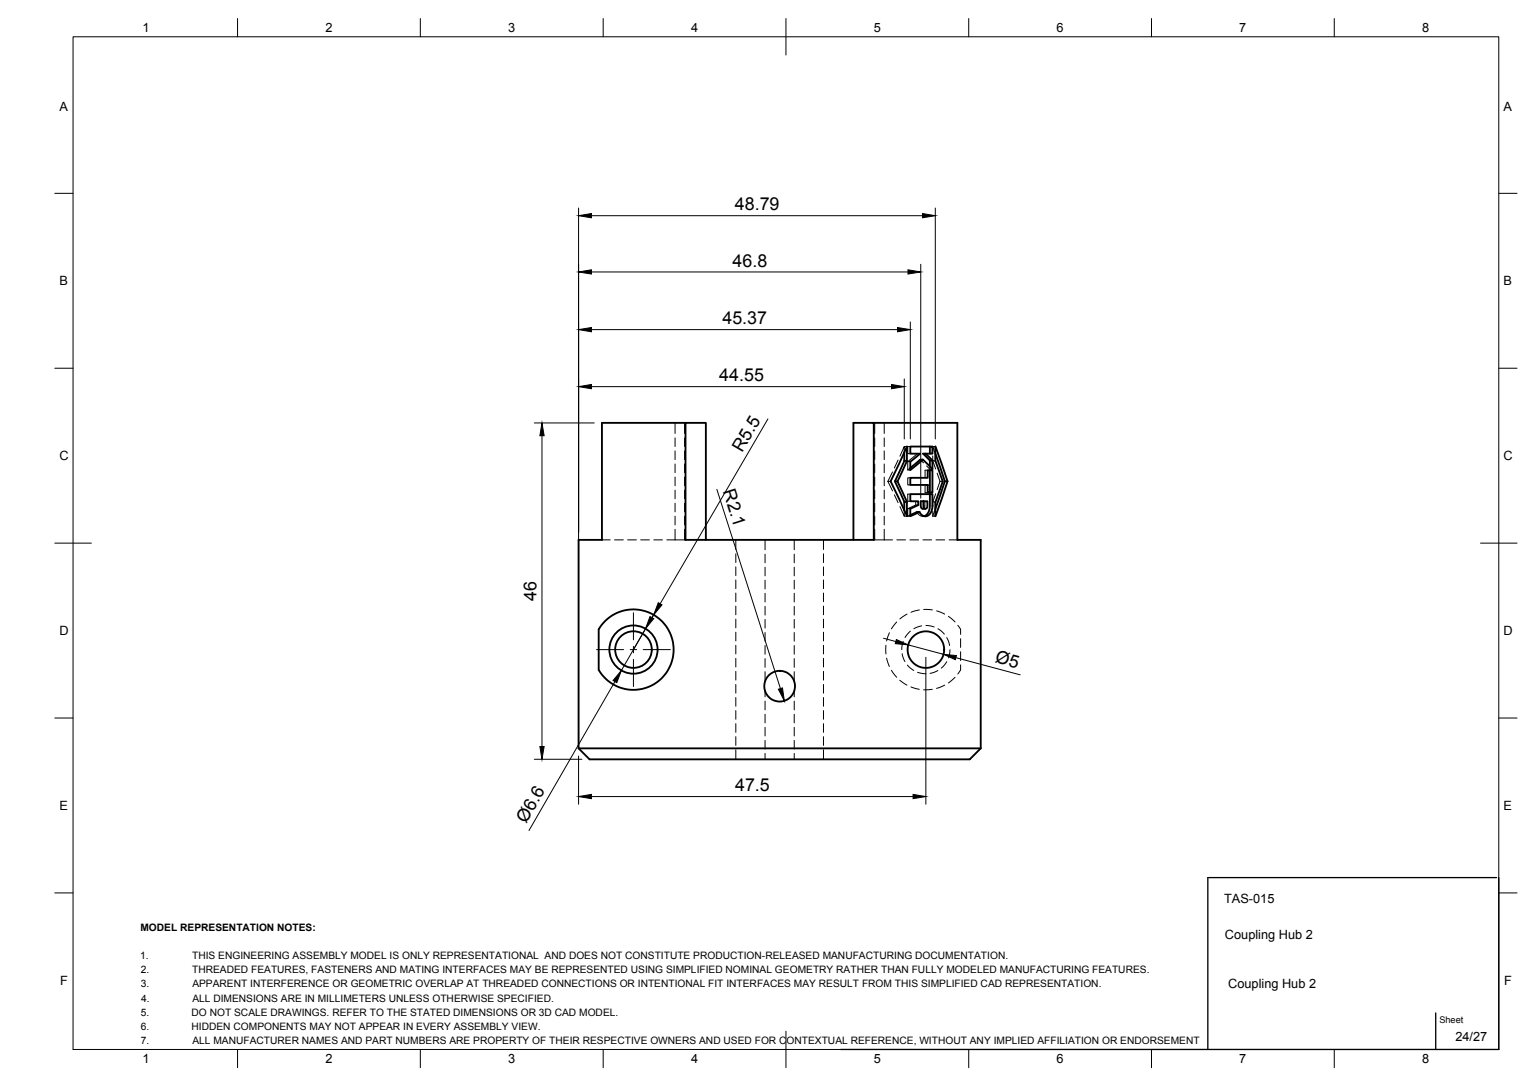
ISO-10303-21;
HEADER;
/* Generated by software containing ST-Developer
 * from STEP Tools, Inc. (www.steptools.com) 
 */

FILE_DESCRIPTION(
/* description */ ('STEP AP214'),
/* implementation_level */ '2;1');

FILE_NAME(
/* name */ 'Coupling Hub 2.step',
/* time_stamp */ '2026-11-15T14:49:54-08:00',
/* author */ (''),
/* organization */ (''),
/* preprocessor_version */ 'ST-DEVELOPER v20.2',
/* originating_system */ 'Autodesk Translation Framework v15.17.0.0',
/* authorisation */ '');

FILE_SCHEMA (('AUTOMOTIVE_DESIGN { 1 0 10303 214 3 1 1 }'));
ENDSEC;

DATA;
#10=MECHANICAL_DESIGN_GEOMETRIC_PRESENTATION_REPRESENTATION('',(#1119,#1120),#66721);
#374=B_SPLINE_CURVE_WITH_KNOTS('',3,(#64255,#64256,#64257,#64258,#64259,
#64260,#64261,#64262,#64263,#64264,#64265,#64266,#64267,#64268,#64269,#64270,
#64271,#64272),.UNSPECIFIED.,.F.,.F.,(4,2,2,2,2,2,2,2,4),(0.567634871268155,
0.624046753014798,0.75751040349095,0.849653931021769,0.941797458552588,
1.03394098608341,1.12608451361423,1.25954816409038,1.39301181456653),
 .UNSPECIFIED.);
#375=B_SPLINE_CURVE_WITH_KNOTS('',3,(#64273,#64274,#64275,#64276,#64277,
#64278,#64279,#64280,#64281,#64282,#64283,#64284,#64285,#64286,#64287,#64288,
#64289,#64290,#64291,#64292,#64293,#64294,#64295,#64296,#64297),
 .UNSPECIFIED.,.F.,.F.,(4,2,2,2,2,3,2,2,2,2,2,4),(1.39301181456653,1.54288207354412,
1.6927523325217,1.78817362481344,1.83588427095931,1.88359491710518,1.93130556325105,
1.97901620939691,2.07443750168865,2.22430776066624,2.37417801964382,2.45122978837333),
 .UNSPECIFIED.);
#376=B_SPLINE_CURVE_WITH_KNOTS('',3,(#64301,#64302,#64303,#64304,#64305,
#64306,#64307,#64308,#64309,#64310,#64311,#64312,#64313,#64314,#64315,#64316,
#64317,#64318,#64319,#64320,#64321,#64322,#64323,#64324,#64325,#64326,#64327,
#64328,#64329,#64330),.UNSPECIFIED.,.F.,.F.,(4,2,2,2,2,2,2,2,2,2,2,2,2,
2,4),(-3.98325608634761,-3.86919217467992,-3.49972652065679,-3.13026086663367,
-2.85088285941717,-2.57150485220067,-2.36940240571059,-2.16729995922052,
-1.96519751273044,-1.76309506624036,-1.48371705902386,-1.20433905180736,
-0.83487339778424,-0.465407743761119,-0.35134383209342),.UNSPECIFIED.);
#377=B_SPLINE_CURVE_WITH_KNOTS('',3,(#64366,#64367,#64368,#64369,#64370,
#64371,#64372,#64373,#64374,#64375,#64376,#64377,#64378,#64379,#64380,#64381,
#64382,#64383,#64384,#64385,#64386,#64387,#64388,#64389,#64390,#64391,#64392,
#64393,#64394,#64395),.UNSPECIFIED.,.F.,.F.,(4,2,2,2,2,2,2,2,2,2,2,2,2,
2,4),(-3.98325608634761,-3.86919217467992,-3.49972652065679,-3.13026086663367,
-2.85088285941717,-2.57150485220067,-2.36940240571059,-2.16729995922052,
-1.96519751273044,-1.76309506624036,-1.48371705902386,-1.20433905180736,
-0.83487339778424,-0.465407743761118,-0.35134383209342),.UNSPECIFIED.);
#378=B_SPLINE_CURVE_WITH_KNOTS('',3,(#64412,#64413,#64414,#64415,#64416,
#64417,#64418,#64419,#64420,#64421,#64422,#64423,#64424,#64425,#64426,#64427,
#64428,#64429,#64430,#64431,#64432,#64433,#64434,#64435,#64436,#64437,#64438,
#64439),.UNSPECIFIED.,.F.,.F.,(4,2,2,2,2,2,2,2,2,2,2,2,2,4),(0.490583102538645,
0.624046753014798,0.75751040349095,0.849653931021769,0.941797458552588,
1.03394098608341,1.12608451361423,1.25954816409038,1.39301181456653,1.54288207354412,
1.6927523325217,1.78817362481344,1.83588427095931,1.88359491710518),
 .UNSPECIFIED.);
#379=B_SPLINE_CURVE_WITH_KNOTS('',3,(#64440,#64441,#64442,#64443,#64444,
#64445,#64446,#64447,#64448,#64449,#64450,#64451),.UNSPECIFIED.,.F.,.F.,
(4,2,2,2,2,4),(0.,0.0477106461458692,0.0954212922917384,0.190842584583477,
0.340712843561061,0.490583102538645),.UNSPECIFIED.);
#380=B_SPLINE_CURVE_WITH_KNOTS('',3,(#64523,#64524,#64525,#64526,#64527,
#64528),.UNSPECIFIED.,.F.,.F.,(4,2,4),(0.575736753726219,0.638728583590876,
0.701720413455533),.UNSPECIFIED.);
#381=B_SPLINE_CURVE_WITH_KNOTS('',3,(#64534,#64535,#64536,#64537,#64538,
#64539,#64540),.UNSPECIFIED.,.F.,.F.,(4,3,4),(-0.0629918298646558,0.,0.0629918298646566),
 .UNSPECIFIED.);
#382=B_SPLINE_CURVE_WITH_KNOTS('',3,(#64547,#64548,#64549,#64550,#64551,
#64552,#64553,#64554,#64555,#64556,#64557,#64558,#64559,#64560,#64561,#64562,
#64563,#64564),.UNSPECIFIED.,.F.,.F.,(4,2,2,2,2,2,2,2,4),(0.,0.0151927838523538,
0.0303855677047076,0.0455818431537581,0.0607781186028086,0.0759788205112384,
0.0911795224196683,0.106372746681134,0.1215659709426),.UNSPECIFIED.);
#383=B_SPLINE_CURVE_WITH_KNOTS('',3,(#64575,#64576,#64577,#64578,#64579,
#64580,#64581,#64582,#64583,#64584,#64585,#64586,#64587,#64588,#64589,#64590,
#64591,#64592),.UNSPECIFIED.,.F.,.F.,(4,2,2,2,2,2,2,2,4),(0.316549052084077,
0.395686269484847,0.474823486885617,0.553960795526886,0.633098104168155,
0.712235412809424,0.791372721450692,0.870509938851462,0.949647156252232),
 .UNSPECIFIED.);
#384=B_SPLINE_CURVE_WITH_KNOTS('',3,(#64594,#64595,#64596,#64597,#64598,
#64599,#64600,#64601,#64602,#64603,#64604,#64605,#64606,#64607,#64608,#64609,
#64610,#64611,#64612,#64613,#64614,#64615,#64616,#64617,#64618,#64619,#64620,
#64621,#64622,#64623,#64624,#64625,#64626,#64627,#64628,#64629,#64630,#64631,
#64632,#64633,#64634,#64635,#64636,#64637,#64638,#64639,#64640,#64641,#64642,
#64643,#64644,#64645,#64646,#64647,#64648,#64649,#64650,#64651,#64652,#64653,
#64654),.UNSPECIFIED.,.F.,.F.,(4,3,3,3,3,3,3,3,3,3,3,3,3,3,3,3,3,3,3,3,
4),(0.,0.0530381009639862,0.106881832368641,0.160741065532074,0.214029097090197,
0.25,0.302729149752815,0.356241665072322,0.409762788184605,0.462708186762728,
0.5,0.552255845605983,0.60528221172878,0.6583187251977,0.710788396881531,
0.75,0.802421738286104,0.855626872469095,0.908846463732818,0.961502691977757,
1.),.UNSPECIFIED.);
#385=B_SPLINE_CURVE_WITH_KNOTS('',3,(#64655,#64656,#64657,#64658,#64659,
#64660,#64661,#64662,#64663,#64664),.UNSPECIFIED.,.F.,.F.,(4,2,2,2,4),(0.949647156252232,
1.028784373653,1.10792159105377,1.18705889969504,1.26619620833631),
 .UNSPECIFIED.);
#386=B_SPLINE_CURVE_WITH_KNOTS('',3,(#64719,#64720,#64721,#64722,#64723,
#64724,#64725,#64726,#64727,#64728,#64729,#64730,#64731,#64732,#64733,#64734),
 .UNSPECIFIED.,.F.,.F.,(4,2,2,2,2,2,2,4),(-0.779703847201594,-0.757646703299412,
-0.7035492015768,-0.649451699854188,-0.595298023055894,-0.5411443462576,
-0.487035463795603,-0.432926581333605),.UNSPECIFIED.);
#387=B_SPLINE_CURVE_WITH_KNOTS('',3,(#64957,#64958,#64959,#64960,#64961,
#64962,#64963,#64964,#64965,#64966,#64967,#64968,#64969,#64970,#64971,#64972),
 .UNSPECIFIED.,.F.,.F.,(4,2,2,2,2,2,2,4),(0.432932407296797,0.487041759940904,
0.541151112585012,0.595306935250484,0.649462757915956,0.703560301016107,
0.757657844116259,0.779715370662846),.UNSPECIFIED.);
#388=B_SPLINE_CURVE_WITH_KNOTS('',3,(#65004,#65005,#65006,#65007,#65008,
#65009,#65010,#65011,#65012,#65013,#65014,#65015,#65016,#65017,#65018,#65019,
#65020,#65021),.UNSPECIFIED.,.F.,.F.,(4,2,2,2,2,2,2,2,4),(0.121566783856533,
0.136760015420318,0.151953246984103,0.167154235901664,0.182355224819225,
0.19755162162294,0.212748018426654,0.22794079306986,0.243133567713066),
 .UNSPECIFIED.);
#553=CONICAL_SURFACE('',#28005,26.75,0.785398163397448);
#554=CONICAL_SURFACE('',#28068,26.75,0.785398163397448);
#658=ELLIPSE('',#28121,54.9999999419771,27.4999999445285);
#659=ELLIPSE('',#28122,55.000000033545,27.5000000336033);
#660=ELLIPSE('',#28123,54.9999999899496,27.4999999902495);
#661=ELLIPSE('',#28124,55.0000000182334,27.5000000177256);
#662=ELLIPSE('',#28125,32.156845610475,27.5);
#663=ELLIPSE('',#28131,33.1709935839343,27.5);
#664=ELLIPSE('',#28132,55.0000000634487,27.5000000626689);
#665=ELLIPSE('',#28133,54.9999999927228,27.4999999930211);
#666=ELLIPSE('',#28134,54.9999999529142,27.4999999544911);
#667=ELLIPSE('',#28135,54.999999883306,27.4999998869508);
#668=ELLIPSE('',#28150,31.5721756903194,27.);
#669=ELLIPSE('',#28153,31.5721756902846,27.);
#670=ELLIPSE('',#28166,32.567884609681,27.);
#671=ELLIPSE('',#28169,54.0000000152791,27.00000001486);
#672=ELLIPSE('',#28170,53.9999998552686,26.9999998599516);
#673=ELLIPSE('',#28171,53.9999996954935,26.9999997042733);
#674=ELLIPSE('',#28172,54.0000000102257,27.0000000099676);
#675=ELLIPSE('',#28181,54.0000000020546,27.0000000020822);
#676=ELLIPSE('',#28183,53.9999999941722,26.9999999944392);
#677=ELLIPSE('',#28186,54.0000000784931,27.0000000775048);
#678=ELLIPSE('',#28188,54.0000000505798,27.0000000505259);
#1057=SHAPE_REPRESENTATION_RELATIONSHIP('SRR','None',#66920,#1088);
#1088=ADVANCED_BREP_SHAPE_REPRESENTATION('',(#1154,#1155),#66711);
#1119=STYLED_ITEM('',(#67095),#1154);
#1120=STYLED_ITEM('',(#67095),#1155);
#1154=MANIFOLD_SOLID_BREP('Body1',#25685);
#1155=MANIFOLD_SOLID_BREP('Body2',#25686);
#1408=FACE_BOUND('',#5046,.T.);
#1409=FACE_BOUND('',#5047,.T.);
#1410=FACE_BOUND('',#5052,.T.);
#1411=FACE_BOUND('',#5055,.T.);
#1412=FACE_BOUND('',#5058,.T.);
#1413=FACE_BOUND('',#5060,.T.);
#1414=FACE_BOUND('',#5064,.T.);
#1415=FACE_BOUND('',#5068,.T.);
#1416=FACE_BOUND('',#5071,.T.);
#1417=FACE_BOUND('',#5073,.T.);
#1418=FACE_BOUND('',#5096,.T.);
#1419=FACE_BOUND('',#5097,.T.);
#1420=FACE_BOUND('',#5098,.T.);
#1421=FACE_BOUND('',#5099,.T.);
#1422=FACE_BOUND('',#5100,.T.);
#1423=FACE_BOUND('',#5101,.T.);
#1424=FACE_BOUND('',#5102,.T.);
#1425=FACE_BOUND('',#5103,.T.);
#1426=FACE_BOUND('',#5153,.T.);
#2055=PLANE('',#28002);
#2056=PLANE('',#28007);
#2057=PLANE('',#28012);
#2058=PLANE('',#28035);
#2059=PLANE('',#28038);
#2060=PLANE('',#28043);
#2061=PLANE('',#28047);
#2062=PLANE('',#28048);
#2063=PLANE('',#28052);
#2064=PLANE('',#28058);
#2065=PLANE('',#28062);
#2066=PLANE('',#28063);
#2067=PLANE('',#28064);
#2068=PLANE('',#28070);
#2069=PLANE('',#28090);
#2070=PLANE('',#28091);
#2071=PLANE('',#28092);
#2072=PLANE('',#28093);
#2073=PLANE('',#28094);
#2074=PLANE('',#28095);
#2075=PLANE('',#28108);
#2076=PLANE('',#28110);
#2077=PLANE('',#28141);
#2078=PLANE('',#28142);
#2079=PLANE('',#28143);
#2080=PLANE('',#28144);
#2081=PLANE('',#28145);
#2082=PLANE('',#28146);
#2083=PLANE('',#28147);
#2084=PLANE('',#28148);
#2085=PLANE('',#28149);
#2086=PLANE('',#28151);
#2087=PLANE('',#28152);
#2088=PLANE('',#28154);
#2089=PLANE('',#28155);
#2090=PLANE('',#28157);
#2091=PLANE('',#28159);
#2092=PLANE('',#28160);
#2093=PLANE('',#28162);
#2094=PLANE('',#28163);
#2095=PLANE('',#28165);
#2096=PLANE('',#28173);
#2097=PLANE('',#28174);
#2098=PLANE('',#28175);
#2099=PLANE('',#28176);
#2100=PLANE('',#28177);
#2101=PLANE('',#28178);
#2102=PLANE('',#28179);
#2103=PLANE('',#28180);
#2104=PLANE('',#28182);
#2105=PLANE('',#28184);
#2106=PLANE('',#28185);
#2107=PLANE('',#28187);
#2108=PLANE('',#28190);
#2109=PLANE('',#28192);
#2110=PLANE('',#28193);
#2111=PLANE('',#28196);
#2112=PLANE('',#28197);
#2113=PLANE('',#28199);
#2114=PLANE('',#28200);
#2115=PLANE('',#28202);
#2116=PLANE('',#28203);
#2117=PLANE('',#28205);
#2118=PLANE('',#28207);
#3353=FACE_OUTER_BOUND('',#5035,.T.);
#3354=FACE_OUTER_BOUND('',#5036,.T.);
#3355=FACE_OUTER_BOUND('',#5037,.T.);
#3356=FACE_OUTER_BOUND('',#5038,.T.);
#3357=FACE_OUTER_BOUND('',#5039,.T.);
#3358=FACE_OUTER_BOUND('',#5040,.T.);
#3359=FACE_OUTER_BOUND('',#5041,.T.);
#3360=FACE_OUTER_BOUND('',#5042,.T.);
#3361=FACE_OUTER_BOUND('',#5043,.T.);
#3362=FACE_OUTER_BOUND('',#5044,.T.);
#3363=FACE_OUTER_BOUND('',#5045,.T.);
#3364=FACE_OUTER_BOUND('',#5048,.T.);
#3365=FACE_OUTER_BOUND('',#5049,.T.);
#3366=FACE_OUTER_BOUND('',#5050,.T.);
#3367=FACE_OUTER_BOUND('',#5051,.T.);
#3368=FACE_OUTER_BOUND('',#5053,.T.);
#3369=FACE_OUTER_BOUND('',#5054,.T.);
#3370=FACE_OUTER_BOUND('',#5056,.T.);
#3371=FACE_OUTER_BOUND('',#5057,.T.);
#3372=FACE_OUTER_BOUND('',#5059,.T.);
#3373=FACE_OUTER_BOUND('',#5061,.T.);
#3374=FACE_OUTER_BOUND('',#5062,.T.);
#3375=FACE_OUTER_BOUND('',#5063,.T.);
#3376=FACE_OUTER_BOUND('',#5065,.T.);
#3377=FACE_OUTER_BOUND('',#5066,.T.);
#3378=FACE_OUTER_BOUND('',#5067,.T.);
#3379=FACE_OUTER_BOUND('',#5069,.T.);
#3380=FACE_OUTER_BOUND('',#5070,.T.);
#3381=FACE_OUTER_BOUND('',#5072,.T.);
#3382=FACE_OUTER_BOUND('',#5074,.T.);
#3383=FACE_OUTER_BOUND('',#5075,.T.);
#3384=FACE_OUTER_BOUND('',#5076,.T.);
#3385=FACE_OUTER_BOUND('',#5077,.T.);
#3386=FACE_OUTER_BOUND('',#5078,.T.);
#3387=FACE_OUTER_BOUND('',#5079,.T.);
#3388=FACE_OUTER_BOUND('',#5080,.T.);
#3389=FACE_OUTER_BOUND('',#5081,.T.);
#3390=FACE_OUTER_BOUND('',#5082,.T.);
#3391=FACE_OUTER_BOUND('',#5083,.T.);
#3392=FACE_OUTER_BOUND('',#5084,.T.);
#3393=FACE_OUTER_BOUND('',#5085,.T.);
#3394=FACE_OUTER_BOUND('',#5086,.T.);
#3395=FACE_OUTER_BOUND('',#5087,.T.);
#3396=FACE_OUTER_BOUND('',#5088,.T.);
#3397=FACE_OUTER_BOUND('',#5089,.T.);
#3398=FACE_OUTER_BOUND('',#5090,.T.);
#3399=FACE_OUTER_BOUND('',#5091,.T.);
#3400=FACE_OUTER_BOUND('',#5092,.T.);
#3401=FACE_OUTER_BOUND('',#5093,.T.);
#3402=FACE_OUTER_BOUND('',#5094,.T.);
#3403=FACE_OUTER_BOUND('',#5095,.T.);
#3404=FACE_OUTER_BOUND('',#5104,.T.);
#3405=FACE_OUTER_BOUND('',#5105,.T.);
#3406=FACE_OUTER_BOUND('',#5106,.T.);
#3407=FACE_OUTER_BOUND('',#5107,.T.);
#3408=FACE_OUTER_BOUND('',#5108,.T.);
#3409=FACE_OUTER_BOUND('',#5109,.T.);
#3410=FACE_OUTER_BOUND('',#5110,.T.);
#3411=FACE_OUTER_BOUND('',#5111,.T.);
#3412=FACE_OUTER_BOUND('',#5112,.T.);
#3413=FACE_OUTER_BOUND('',#5113,.T.);
#3414=FACE_OUTER_BOUND('',#5114,.T.);
#3415=FACE_OUTER_BOUND('',#5115,.T.);
#3416=FACE_OUTER_BOUND('',#5116,.T.);
#3417=FACE_OUTER_BOUND('',#5117,.T.);
#3418=FACE_OUTER_BOUND('',#5118,.T.);
#3419=FACE_OUTER_BOUND('',#5119,.T.);
#3420=FACE_OUTER_BOUND('',#5120,.T.);
#3421=FACE_OUTER_BOUND('',#5121,.T.);
#3422=FACE_OUTER_BOUND('',#5122,.T.);
#3423=FACE_OUTER_BOUND('',#5123,.T.);
#3424=FACE_OUTER_BOUND('',#5124,.T.);
#3425=FACE_OUTER_BOUND('',#5125,.T.);
#3426=FACE_OUTER_BOUND('',#5126,.T.);
#3427=FACE_OUTER_BOUND('',#5127,.T.);
#3428=FACE_OUTER_BOUND('',#5128,.T.);
#3429=FACE_OUTER_BOUND('',#5129,.T.);
#3430=FACE_OUTER_BOUND('',#5130,.T.);
#3431=FACE_OUTER_BOUND('',#5131,.T.);
#3432=FACE_OUTER_BOUND('',#5132,.T.);
#3433=FACE_OUTER_BOUND('',#5133,.T.);
#3434=FACE_OUTER_BOUND('',#5134,.T.);
#3435=FACE_OUTER_BOUND('',#5135,.T.);
#3436=FACE_OUTER_BOUND('',#5136,.T.);
#3437=FACE_OUTER_BOUND('',#5137,.T.);
#3438=FACE_OUTER_BOUND('',#5138,.T.);
#3439=FACE_OUTER_BOUND('',#5139,.T.);
#3440=FACE_OUTER_BOUND('',#5140,.T.);
#3441=FACE_OUTER_BOUND('',#5141,.T.);
#3442=FACE_OUTER_BOUND('',#5142,.T.);
#3443=FACE_OUTER_BOUND('',#5143,.T.);
#3444=FACE_OUTER_BOUND('',#5144,.T.);
#3445=FACE_OUTER_BOUND('',#5145,.T.);
#3446=FACE_OUTER_BOUND('',#5146,.T.);
#3447=FACE_OUTER_BOUND('',#5147,.T.);
#3448=FACE_OUTER_BOUND('',#5148,.T.);
#3449=FACE_OUTER_BOUND('',#5149,.T.);
#3450=FACE_OUTER_BOUND('',#5150,.T.);
#3451=FACE_OUTER_BOUND('',#5151,.T.);
#3452=FACE_OUTER_BOUND('',#5152,.T.);
#5035=EDGE_LOOP('',(#22080,#22081,#22082,#22083));
#5036=EDGE_LOOP('',(#22084,#22085,#22086,#22087));
#5037=EDGE_LOOP('',(#22088,#22089,#22090,#22091));
#5038=EDGE_LOOP('',(#22092,#22093,#22094,#22095));
#5039=EDGE_LOOP('',(#22096,#22097,#22098,#22099));
#5040=EDGE_LOOP('',(#22100,#22101,#22102,#22103));
#5041=EDGE_LOOP('',(#22104,#22105,#22106,#22107));
#5042=EDGE_LOOP('',(#22108,#22109,#22110,#22111));
#5043=EDGE_LOOP('',(#22112,#22113,#22114,#22115));
#5044=EDGE_LOOP('',(#22116,#22117,#22118,#22119));
#5045=EDGE_LOOP('',(#22120,#22121,#22122,#22123,#22124,#22125,#22126,#22127,
#22128,#22129,#22130,#22131));
#5046=EDGE_LOOP('',(#22132,#22133));
#5047=EDGE_LOOP('',(#22134,#22135));
#5048=EDGE_LOOP('',(#22136,#22137,#22138,#22139));
#5049=EDGE_LOOP('',(#22140,#22141,#22142,#22143,#22144,#22145,#22146,#22147,
#22148,#22149,#22150,#22151));
#5050=EDGE_LOOP('',(#22152,#22153,#22154,#22155,#22156));
#5051=EDGE_LOOP('',(#22157,#22158));
#5052=EDGE_LOOP('',(#22159));
#5053=EDGE_LOOP('',(#22160,#22161,#22162,#22163));
#5054=EDGE_LOOP('',(#22164));
#5055=EDGE_LOOP('',(#22165));
#5056=EDGE_LOOP('',(#22166,#22167,#22168,#22169));
#5057=EDGE_LOOP('',(#22170,#22171,#22172,#22173,#22174));
#5058=EDGE_LOOP('',(#22175));
#5059=EDGE_LOOP('',(#22176,#22177,#22178,#22179,#22180));
#5060=EDGE_LOOP('',(#22181));
#5061=EDGE_LOOP('',(#22182,#22183));
#5062=EDGE_LOOP('',(#22184,#22185));
#5063=EDGE_LOOP('',(#22186,#22187,#22188,#22189,#22190));
#5064=EDGE_LOOP('',(#22191));
#5065=EDGE_LOOP('',(#22192,#22193,#22194,#22195,#22196));
#5066=EDGE_LOOP('',(#22197,#22198,#22199,#22200));
#5067=EDGE_LOOP('',(#22201));
#5068=EDGE_LOOP('',(#22202));
#5069=EDGE_LOOP('',(#22203,#22204,#22205,#22206));
#5070=EDGE_LOOP('',(#22207,#22208));
#5071=EDGE_LOOP('',(#22209));
#5072=EDGE_LOOP('',(#22210,#22211,#22212,#22213,#22214));
#5073=EDGE_LOOP('',(#22215));
#5074=EDGE_LOOP('',(#22216,#22217,#22218,#22219,#22220,#22221,#22222,#22223));
#5075=EDGE_LOOP('',(#22224,#22225,#22226,#22227));
#5076=EDGE_LOOP('',(#22228,#22229,#22230,#22231,#22232,#22233,#22234,#22235,
#22236,#22237,#22238,#22239,#22240,#22241,#22242,#22243));
#5077=EDGE_LOOP('',(#22244,#22245,#22246,#22247,#22248,#22249));
#5078=EDGE_LOOP('',(#22250,#22251,#22252,#22253,#22254,#22255));
#5079=EDGE_LOOP('',(#22256,#22257,#22258,#22259));
#5080=EDGE_LOOP('',(#22260,#22261,#22262,#22263,#22264,#22265,#22266,#22267,
#22268,#22269,#22270,#22271,#22272,#22273));
#5081=EDGE_LOOP('',(#22274,#22275,#22276,#22277));
#5082=EDGE_LOOP('',(#22278,#22279,#22280,#22281));
#5083=EDGE_LOOP('',(#22282,#22283,#22284,#22285,#22286));
#5084=EDGE_LOOP('',(#22287,#22288,#22289,#22290));
#5085=EDGE_LOOP('',(#22291,#22292,#22293,#22294));
#5086=EDGE_LOOP('',(#22295,#22296,#22297,#22298));
#5087=EDGE_LOOP('',(#22299,#22300,#22301,#22302));
#5088=EDGE_LOOP('',(#22303,#22304,#22305,#22306));
#5089=EDGE_LOOP('',(#22307,#22308,#22309,#22310));
#5090=EDGE_LOOP('',(#22311,#22312,#22313,#22314));
#5091=EDGE_LOOP('',(#22315,#22316,#22317,#22318));
#5092=EDGE_LOOP('',(#22319,#22320,#22321,#22322));
#5093=EDGE_LOOP('',(#22323,#22324,#22325,#22326));
#5094=EDGE_LOOP('',(#22327,#22328,#22329,#22330));
#5095=EDGE_LOOP('',(#22331,#22332,#22333,#22334,#22335,#22336,#22337,#22338,
#22339,#22340,#22341,#22342));
#5096=EDGE_LOOP('',(#22343,#22344));
#5097=EDGE_LOOP('',(#22345,#22346,#22347,#22348,#22349,#22350,#22351,#22352,
#22353));
#5098=EDGE_LOOP('',(#22354,#22355,#22356,#22357,#22358,#22359,#22360,#22361));
#5099=EDGE_LOOP('',(#22362,#22363,#22364));
#5100=EDGE_LOOP('',(#22365,#22366));
#5101=EDGE_LOOP('',(#22367,#22368,#22369,#22370,#22371,#22372));
#5102=EDGE_LOOP('',(#22373,#22374,#22375,#22376,#22377,#22378,#22379,#22380,
#22381,#22382,#22383));
#5103=EDGE_LOOP('',(#22384,#22385,#22386,#22387,#22388,#22389));
#5104=EDGE_LOOP('',(#22390,#22391,#22392,#22393,#22394,#22395,#22396,#22397));
#5105=EDGE_LOOP('',(#22398,#22399,#22400,#22401));
#5106=EDGE_LOOP('',(#22402,#22403,#22404,#22405));
#5107=EDGE_LOOP('',(#22406,#22407,#22408,#22409));
#5108=EDGE_LOOP('',(#22410,#22411,#22412,#22413));
#5109=EDGE_LOOP('',(#22414,#22415,#22416,#22417));
#5110=EDGE_LOOP('',(#22418,#22419,#22420,#22421));
#5111=EDGE_LOOP('',(#22422,#22423,#22424,#22425));
#5112=EDGE_LOOP('',(#22426,#22427,#22428,#22429));
#5113=EDGE_LOOP('',(#22430,#22431,#22432,#22433));
#5114=EDGE_LOOP('',(#22434,#22435,#22436,#22437));
#5115=EDGE_LOOP('',(#22438,#22439,#22440,#22441));
#5116=EDGE_LOOP('',(#22442,#22443,#22444,#22445));
#5117=EDGE_LOOP('',(#22446,#22447,#22448,#22449));
#5118=EDGE_LOOP('',(#22450,#22451,#22452,#22453));
#5119=EDGE_LOOP('',(#22454,#22455,#22456,#22457));
#5120=EDGE_LOOP('',(#22458,#22459,#22460,#22461));
#5121=EDGE_LOOP('',(#22462,#22463,#22464,#22465));
#5122=EDGE_LOOP('',(#22466,#22467,#22468,#22469));
#5123=EDGE_LOOP('',(#22470,#22471,#22472,#22473));
#5124=EDGE_LOOP('',(#22474,#22475,#22476,#22477,#22478,#22479,#22480,#22481,
#22482,#22483,#22484));
#5125=EDGE_LOOP('',(#22485,#22486,#22487,#22488,#22489,#22490));
#5126=EDGE_LOOP('',(#22491,#22492,#22493,#22494));
#5127=EDGE_LOOP('',(#22495,#22496,#22497,#22498));
#5128=EDGE_LOOP('',(#22499,#22500,#22501,#22502));
#5129=EDGE_LOOP('',(#22503,#22504,#22505,#22506));
#5130=EDGE_LOOP('',(#22507,#22508,#22509,#22510));
#5131=EDGE_LOOP('',(#22511,#22512,#22513,#22514));
#5132=EDGE_LOOP('',(#22515,#22516,#22517,#22518));
#5133=EDGE_LOOP('',(#22519,#22520,#22521,#22522));
#5134=EDGE_LOOP('',(#22523,#22524,#22525,#22526));
#5135=EDGE_LOOP('',(#22527,#22528,#22529,#22530));
#5136=EDGE_LOOP('',(#22531,#22532,#22533,#22534));
#5137=EDGE_LOOP('',(#22535,#22536,#22537,#22538));
#5138=EDGE_LOOP('',(#22539,#22540,#22541,#22542,#22543,#22544));
#5139=EDGE_LOOP('',(#22545,#22546,#22547,#22548));
#5140=EDGE_LOOP('',(#22549,#22550,#22551,#22552));
#5141=EDGE_LOOP('',(#22553,#22554,#22555,#22556));
#5142=EDGE_LOOP('',(#22557,#22558,#22559,#22560));
#5143=EDGE_LOOP('',(#22561,#22562,#22563,#22564));
#5144=EDGE_LOOP('',(#22565,#22566,#22567,#22568));
#5145=EDGE_LOOP('',(#22569,#22570,#22571,#22572));
#5146=EDGE_LOOP('',(#22573,#22574,#22575,#22576));
#5147=EDGE_LOOP('',(#22577,#22578,#22579,#22580));
#5148=EDGE_LOOP('',(#22581,#22582,#22583,#22584));
#5149=EDGE_LOOP('',(#22585,#22586,#22587,#22588));
#5150=EDGE_LOOP('',(#22589,#22590,#22591,#22592));
#5151=EDGE_LOOP('',(#22593,#22594,#22595,#22596));
#5152=EDGE_LOOP('',(#22597,#22598,#22599,#22600,#22601,#22602,#22603,#22604,
#22605));
#5153=EDGE_LOOP('',(#22606,#22607,#22608,#22609));
#6962=LINE('',#64187,#8951);
#6963=LINE('',#64191,#8952);
#6964=LINE('',#64197,#8953);
#6965=LINE('',#64198,#8954);
#6966=LINE('',#64221,#8955);
#6967=LINE('',#64222,#8956);
#6968=LINE('',#64225,#8957);
#6969=LINE('',#64227,#8958);
#6970=LINE('',#64231,#8959);
#6971=LINE('',#64235,#8960);
#6972=LINE('',#64240,#8961);
#6973=LINE('',#64244,#8962);
#6974=LINE('',#64249,#8963);
#6975=LINE('',#64251,#8964);
#6976=LINE('',#64300,#8965);
#6977=LINE('',#64333,#8966);
#6978=LINE('',#64336,#8967);
#6979=LINE('',#64338,#8968);
#6980=LINE('',#64339,#8969);
#6981=LINE('',#64342,#8970);
#6982=LINE('',#64351,#8971);
#6983=LINE('',#64358,#8972);
#6984=LINE('',#64399,#8973);
#6985=LINE('',#64401,#8974);
#6986=LINE('',#64403,#8975);
#6987=LINE('',#64405,#8976);
#6988=LINE('',#64406,#8977);
#6989=LINE('',#64452,#8978);
#6990=LINE('',#64457,#8979);
#6991=LINE('',#64464,#8980);
#6992=LINE('',#64467,#8981);
#6993=LINE('',#64471,#8982);
#6994=LINE('',#64473,#8983);
#6995=LINE('',#64475,#8984);
#6996=LINE('',#64477,#8985);
#6997=LINE('',#64478,#8986);
#6998=LINE('',#64483,#8987);
#6999=LINE('',#64485,#8988);
#7000=LINE('',#64487,#8989);
#7001=LINE('',#64513,#8990);
#7002=LINE('',#64515,#8991);
#7003=LINE('',#64517,#8992);
#7004=LINE('',#64521,#8993);
#7005=LINE('',#64529,#8994);
#7006=LINE('',#64532,#8995);
#7007=LINE('',#64541,#8996);
#7008=LINE('',#64545,#8997);
#7009=LINE('',#64566,#8998);
#7010=LINE('',#64573,#8999);
#7011=LINE('',#64667,#9000);
#7012=LINE('',#64669,#9001);
#7013=LINE('',#64672,#9002);
#7014=LINE('',#64673,#9003);
#7015=LINE('',#64675,#9004);
#7016=LINE('',#64677,#9005);
#7017=LINE('',#64679,#9006);
#7018=LINE('',#64681,#9007);
#7019=LINE('',#64688,#9008);
#7020=LINE('',#64689,#9009);
#7021=LINE('',#64694,#9010);
#7022=LINE('',#64695,#9011);
#7023=LINE('',#64698,#9012);
#7024=LINE('',#64701,#9013);
#7025=LINE('',#64705,#9014);
#7026=LINE('',#64710,#9015);
#7027=LINE('',#64738,#9016);
#7028=LINE('',#64742,#9017);
#7029=LINE('',#64746,#9018);
#7030=LINE('',#64749,#9019);
#7031=LINE('',#64754,#9020);
#7032=LINE('',#64758,#9021);
#7033=LINE('',#64762,#9022);
#7034=LINE('',#64765,#9023);
#7035=LINE('',#64768,#9024);
#7036=LINE('',#64774,#9025);
#7037=LINE('',#64782,#9026);
#7038=LINE('',#64788,#9027);
#7039=LINE('',#64792,#9028);
#7040=LINE('',#64798,#9029);
#7041=LINE('',#64804,#9030);
#7042=LINE('',#64810,#9031);
#7043=LINE('',#64817,#9032);
#7044=LINE('',#64821,#9033);
#7045=LINE('',#64825,#9034);
#7046=LINE('',#64828,#9035);
#7047=LINE('',#64830,#9036);
#7048=LINE('',#64831,#9037);
#7049=LINE('',#64833,#9038);
#7050=LINE('',#64835,#9039);
#7051=LINE('',#64837,#9040);
#7052=LINE('',#64839,#9041);
#7053=LINE('',#64841,#9042);
#7054=LINE('',#64843,#9043);
#7055=LINE('',#64847,#9044);
#7056=LINE('',#64850,#9045);
#7057=LINE('',#64853,#9046);
#7058=LINE('',#64854,#9047);
#7059=LINE('',#64857,#9048);
#7060=LINE('',#64861,#9049);
#7061=LINE('',#64863,#9050);
#7062=LINE('',#64864,#9051);
#7063=LINE('',#64867,#9052);
#7064=LINE('',#64871,#9053);
#7065=LINE('',#64875,#9054);
#7066=LINE('',#64876,#9055);
#7067=LINE('',#64879,#9056);
#7068=LINE('',#64883,#9057);
#7069=LINE('',#64884,#9058);
#7070=LINE('',#64895,#9059);
#7071=LINE('',#64901,#9060);
#7072=LINE('',#64904,#9061);
#7073=LINE('',#64905,#9062);
#7074=LINE('',#64907,#9063);
#7075=LINE('',#64909,#9064);
#7076=LINE('',#64911,#9065);
#7077=LINE('',#64913,#9066);
#7078=LINE('',#64917,#9067);
#7079=LINE('',#64919,#9068);
#7080=LINE('',#64920,#9069);
#7081=LINE('',#64923,#9070);
#7082=LINE('',#64927,#9071);
#7083=LINE('',#64931,#9072);
#7084=LINE('',#64932,#9073);
#7085=LINE('',#64936,#9074);
#7086=LINE('',#64942,#9075);
#7087=LINE('',#64945,#9076);
#7088=LINE('',#64948,#9077);
#7089=LINE('',#64949,#9078);
#7090=LINE('',#64952,#9079);
#7091=LINE('',#64956,#9080);
#7092=LINE('',#64975,#9081);
#7093=LINE('',#64976,#9082);
#7094=LINE('',#64979,#9083);
#7095=LINE('',#64982,#9084);
#7096=LINE('',#64985,#9085);
#7097=LINE('',#64986,#9086);
#7098=LINE('',#64989,#9087);
#7099=LINE('',#64993,#9088);
#7100=LINE('',#64994,#9089);
#7101=LINE('',#64997,#9090);
#7102=LINE('',#65000,#9091);
#7103=LINE('',#65003,#9092);
#7104=LINE('',#65023,#9093);
#8951=VECTOR('',#34159,1000.);
#8952=VECTOR('',#34162,1000.);
#8953=VECTOR('',#34169,1000.);
#8954=VECTOR('',#34170,1000.);
#8955=VECTOR('',#34195,1000.);
#8956=VECTOR('',#34196,1000.);
#8957=VECTOR('',#34199,1000.);
#8958=VECTOR('',#34200,1000.);
#8959=VECTOR('',#34205,1000.);
#8960=VECTOR('',#34210,1000.);
#8961=VECTOR('',#34217,1000.);
#8962=VECTOR('',#34222,1000.);
#8963=VECTOR('',#34229,1000.);
#8964=VECTOR('',#34230,1000.);
#8965=VECTOR('',#34233,1000.);
#8966=VECTOR('',#34236,1000.);
#8967=VECTOR('',#34239,1000.);
#8968=VECTOR('',#34242,1000.);
#8969=VECTOR('',#34243,1000.);
#8970=VECTOR('',#34246,2.5);
#8971=VECTOR('',#34259,3.3);
#8972=VECTOR('',#34268,2.5);
#8973=VECTOR('',#34281,1000.);
#8974=VECTOR('',#34282,1000.);
#8975=VECTOR('',#34283,1000.);
#8976=VECTOR('',#34284,1000.);
#8977=VECTOR('',#34285,1000.);
#8978=VECTOR('',#34290,2.5);
#8979=VECTOR('',#34295,2.5);
#8980=VECTOR('',#34304,3.3);
#8981=VECTOR('',#34309,1000.);
#8982=VECTOR('',#34312,1000.);
#8983=VECTOR('',#34313,1000.);
#8984=VECTOR('',#34314,1000.);
#8985=VECTOR('',#34315,1000.);
#8986=VECTOR('',#34316,1000.);
#8987=VECTOR('',#34321,1000.);
#8988=VECTOR('',#34322,1000.);
#8989=VECTOR('',#34323,1000.);
#8990=VECTOR('',#34354,1000.);
#8991=VECTOR('',#34355,1000.);
#8992=VECTOR('',#34356,1000.);
#8993=VECTOR('',#34361,1000.);
#8994=VECTOR('',#34362,1000.);
#8995=VECTOR('',#34365,1000.);
#8996=VECTOR('',#34366,1000.);
#8997=VECTOR('',#34369,1000.);
#8998=VECTOR('',#34370,1000.);
#8999=VECTOR('',#34377,2.1);
#9000=VECTOR('',#34380,1000.);
#9001=VECTOR('',#34381,1000.);
#9002=VECTOR('',#34384,1000.);
#9003=VECTOR('',#34385,1000.);
#9004=VECTOR('',#34388,1000.);
#9005=VECTOR('',#34391,1000.);
#9006=VECTOR('',#34394,1000.);
#9007=VECTOR('',#34397,1000.);
#9008=VECTOR('',#34406,1000.);
#9009=VECTOR('',#34407,1000.);
#9010=VECTOR('',#34412,1000.);
#9011=VECTOR('',#34413,1000.);
#9012=VECTOR('',#34416,1000.);
#9013=VECTOR('',#34419,1000.);
#9014=VECTOR('',#34424,1000.);
#9015=VECTOR('',#34431,1000.);
#9016=VECTOR('',#34446,1000.);
#9017=VECTOR('',#34449,1000.);
#9018=VECTOR('',#34452,1000.);
#9019=VECTOR('',#34455,1000.);
#9020=VECTOR('',#34458,1000.);
#9021=VECTOR('',#34461,1000.);
#9022=VECTOR('',#34464,1000.);
#9023=VECTOR('',#34467,1000.);
#9024=VECTOR('',#34468,1000.);
#9025=VECTOR('',#34473,1000.);
#9026=VECTOR('',#34480,1000.);
#9027=VECTOR('',#34485,1000.);
#9028=VECTOR('',#34488,1000.);
#9029=VECTOR('',#34493,1000.);
#9030=VECTOR('',#34498,1000.);
#9031=VECTOR('',#34503,1000.);
#9032=VECTOR('',#34510,1000.);
#9033=VECTOR('',#34513,1000.);
#9034=VECTOR('',#34516,1000.);
#9035=VECTOR('',#34519,1000.);
#9036=VECTOR('',#34522,1000.);
#9037=VECTOR('',#34523,1000.);
#9038=VECTOR('',#34526,1000.);
#9039=VECTOR('',#34529,1000.);
#9040=VECTOR('',#34532,1000.);
#9041=VECTOR('',#34535,1000.);
#9042=VECTOR('',#34538,1000.);
#9043=VECTOR('',#34541,1000.);
#9044=VECTOR('',#34546,1000.);
#9045=VECTOR('',#34549,1000.);
#9046=VECTOR('',#34552,1000.);
#9047=VECTOR('',#34553,1000.);
#9048=VECTOR('',#34556,1000.);
#9049=VECTOR('',#34561,1000.);
#9050=VECTOR('',#34562,1000.);
#9051=VECTOR('',#34563,1000.);
#9052=VECTOR('',#34566,1000.);
#9053=VECTOR('',#34571,1000.);
#9054=VECTOR('',#34576,1000.);
#9055=VECTOR('',#34577,1000.);
#9056=VECTOR('',#34580,1000.);
#9057=VECTOR('',#34585,1000.);
#9058=VECTOR('',#34586,1000.);
#9059=VECTOR('',#34601,1000.);
#9060=VECTOR('',#34606,1000.);
#9061=VECTOR('',#34611,1000.);
#9062=VECTOR('',#34612,1000.);
#9063=VECTOR('',#34615,1000.);
#9064=VECTOR('',#34618,1000.);
#9065=VECTOR('',#34621,1000.);
#9066=VECTOR('',#34624,1000.);
#9067=VECTOR('',#34629,1000.);
#9068=VECTOR('',#34630,1000.);
#9069=VECTOR('',#34631,1000.);
#9070=VECTOR('',#34634,1000.);
#9071=VECTOR('',#34639,1000.);
#9072=VECTOR('',#34644,1000.);
#9073=VECTOR('',#34645,1000.);
#9074=VECTOR('',#34650,1000.);
#9075=VECTOR('',#34659,1000.);
#9076=VECTOR('',#34662,1000.);
#9077=VECTOR('',#34665,1000.);
#9078=VECTOR('',#34666,1000.);
#9079=VECTOR('',#34669,1000.);
#9080=VECTOR('',#34674,1000.);
#9081=VECTOR('',#34677,1000.);
#9082=VECTOR('',#34678,1000.);
#9083=VECTOR('',#34681,1000.);
#9084=VECTOR('',#34684,1000.);
#9085=VECTOR('',#34687,1000.);
#9086=VECTOR('',#34688,1000.);
#9087=VECTOR('',#34691,1000.);
#9088=VECTOR('',#34696,1000.);
#9089=VECTOR('',#34697,1000.);
#9090=VECTOR('',#34700,1000.);
#9091=VECTOR('',#34705,1000.);
#9092=VECTOR('',#34708,1000.);
#9093=VECTOR('',#34711,1000.);
#10357=CIRCLE('',#28003,26.);
#10358=CIRCLE('',#28004,6.);
#10359=CIRCLE('',#28006,27.5);
#10360=CIRCLE('',#28008,13.);
#10361=CIRCLE('',#28009,27.5);
#10362=CIRCLE('',#28010,13.);
#10363=CIRCLE('',#28011,17.5);
#10364=CIRCLE('',#28013,13.);
#10365=CIRCLE('',#28014,27.5);
#10366=CIRCLE('',#28015,13.);
#10367=CIRCLE('',#28016,17.5);
#10368=CIRCLE('',#28018,17.5);
#10369=CIRCLE('',#28020,17.5);
#10370=CIRCLE('',#28022,13.);
#10371=CIRCLE('',#28024,13.);
#10372=CIRCLE('',#28026,13.);
#10373=CIRCLE('',#28028,13.);
#10374=CIRCLE('',#28030,27.5);
#10375=CIRCLE('',#28031,27.5);
#10376=CIRCLE('',#28032,27.5);
#10377=CIRCLE('',#28034,6.);
#10378=CIRCLE('',#28037,2.5);
#10379=CIRCLE('',#28039,5.5);
#10380=CIRCLE('',#28040,3.3);
#10381=CIRCLE('',#28042,3.3);
#10382=CIRCLE('',#28044,2.5);
#10383=CIRCLE('',#28046,2.5);
#10384=CIRCLE('',#28051,5.5);
#10385=CIRCLE('',#28053,2.5);
#10386=CIRCLE('',#28056,2.5);
#10387=CIRCLE('',#28057,2.5);
#10388=CIRCLE('',#28059,3.3);
#10389=CIRCLE('',#28061,3.3);
#10390=CIRCLE('',#28065,6.);
#10391=CIRCLE('',#28066,6.);
#10392=CIRCLE('',#28067,26.);
#10393=CIRCLE('',#28069,27.5);
#10394=CIRCLE('',#28071,27.5);
#10395=CIRCLE('',#28072,13.);
#10396=CIRCLE('',#28073,17.5);
#10397=CIRCLE('',#28074,13.);
#10398=CIRCLE('',#28075,27.5);
#10399=CIRCLE('',#28076,13.);
#10400=CIRCLE('',#28077,17.5);
#10401=CIRCLE('',#28078,13.);
#10402=CIRCLE('',#28079,27.5);
#10403=CIRCLE('',#28080,6.);
#10404=CIRCLE('',#28081,6.);
#10405=CIRCLE('',#28085,27.5);
#10406=CIRCLE('',#28087,2.1);
#10407=CIRCLE('',#28088,2.1);
#10408=CIRCLE('',#28089,2.1);
#10409=CIRCLE('',#28097,13.);
#10410=CIRCLE('',#28099,13.);
#10411=CIRCLE('',#28101,13.);
#10412=CIRCLE('',#28103,17.5);
#10413=CIRCLE('',#28105,17.5);
#10414=CIRCLE('',#28107,13.);
#10415=CIRCLE('',#28109,27.5);
#10416=CIRCLE('',#28111,27.5);
#10417=CIRCLE('',#28113,30.7157076297161);
#10418=CIRCLE('',#28114,30.7139923780105);
#10419=CIRCLE('',#28115,27.5);
#10420=CIRCLE('',#28116,27.5);
#10421=CIRCLE('',#28117,27.5);
#10422=CIRCLE('',#28118,27.5);
#10423=CIRCLE('',#28119,27.5);
#10424=CIRCLE('',#28120,27.5);
#10425=CIRCLE('',#28126,37.5686105496298);
#10426=CIRCLE('',#28127,27.5);
#10427=CIRCLE('',#28128,27.5);
#10428=CIRCLE('',#28129,27.5);
#10429=CIRCLE('',#28130,39.9577086924719);
#10430=CIRCLE('',#28137,27.);
#10431=CIRCLE('',#28138,27.);
#10432=CIRCLE('',#28139,27.);
#10433=CIRCLE('',#28140,27.);
#10434=CIRCLE('',#28156,39.2292319119626);
#10435=CIRCLE('',#28158,27.);
#10436=CIRCLE('',#28161,27.);
#10437=CIRCLE('',#28164,27.);
#10438=CIRCLE('',#28191,30.1550686144397);
#10439=CIRCLE('',#28194,30.1568155811873);
#10440=CIRCLE('',#28198,27.);
#10441=CIRCLE('',#28201,27.);
#10442=CIRCLE('',#28204,27.);
#12411=VERTEX_POINT('',#64185);
#12412=VERTEX_POINT('',#64186);
#12413=VERTEX_POINT('',#64188);
#12414=VERTEX_POINT('',#64190);
#12415=VERTEX_POINT('',#64194);
#12416=VERTEX_POINT('',#64195);
#12417=VERTEX_POINT('',#64200);
#12418=VERTEX_POINT('',#64201);
#12419=VERTEX_POINT('',#64203);
#12420=VERTEX_POINT('',#64205);
#12421=VERTEX_POINT('',#64209);
#12422=VERTEX_POINT('',#64210);
#12423=VERTEX_POINT('',#64212);
#12424=VERTEX_POINT('',#64214);
#12425=VERTEX_POINT('',#64218);
#12426=VERTEX_POINT('',#64219);
#12427=VERTEX_POINT('',#64224);
#12428=VERTEX_POINT('',#64226);
#12429=VERTEX_POINT('',#64230);
#12430=VERTEX_POINT('',#64234);
#12431=VERTEX_POINT('',#64238);
#12432=VERTEX_POINT('',#64242);
#12433=VERTEX_POINT('',#64247);
#12434=VERTEX_POINT('',#64250);
#12435=VERTEX_POINT('',#64253);
#12436=VERTEX_POINT('',#64254);
#12437=VERTEX_POINT('',#64298);
#12438=VERTEX_POINT('',#64299);
#12439=VERTEX_POINT('',#64332);
#12440=VERTEX_POINT('',#64334);
#12441=VERTEX_POINT('',#64341);
#12442=VERTEX_POINT('',#64346);
#12443=VERTEX_POINT('',#64349);
#12444=VERTEX_POINT('',#64353);
#12445=VERTEX_POINT('',#64356);
#12446=VERTEX_POINT('',#64363);
#12447=VERTEX_POINT('',#64364);
#12448=VERTEX_POINT('',#64397);
#12449=VERTEX_POINT('',#64398);
#12450=VERTEX_POINT('',#64400);
#12451=VERTEX_POINT('',#64402);
#12452=VERTEX_POINT('',#64404);
#12453=VERTEX_POINT('',#64407);
#12454=VERTEX_POINT('',#64410);
#12455=VERTEX_POINT('',#64411);
#12456=VERTEX_POINT('',#64454);
#12457=VERTEX_POINT('',#64456);
#12458=VERTEX_POINT('',#64460);
#12459=VERTEX_POINT('',#64463);
#12460=VERTEX_POINT('',#64469);
#12461=VERTEX_POINT('',#64470);
#12462=VERTEX_POINT('',#64472);
#12463=VERTEX_POINT('',#64474);
#12464=VERTEX_POINT('',#64476);
#12465=VERTEX_POINT('',#64480);
#12466=VERTEX_POINT('',#64482);
#12467=VERTEX_POINT('',#64484);
#12468=VERTEX_POINT('',#64486);
#12469=VERTEX_POINT('',#64493);
#12470=VERTEX_POINT('',#64495);
#12471=VERTEX_POINT('',#64497);
#12472=VERTEX_POINT('',#64499);
#12473=VERTEX_POINT('',#64501);
#12474=VERTEX_POINT('',#64503);
#12475=VERTEX_POINT('',#64505);
#12476=VERTEX_POINT('',#64507);
#12477=VERTEX_POINT('',#64510);
#12478=VERTEX_POINT('',#64512);
#12479=VERTEX_POINT('',#64514);
#12480=VERTEX_POINT('',#64516);
#12481=VERTEX_POINT('',#64520);
#12482=VERTEX_POINT('',#64522);
#12483=VERTEX_POINT('',#64531);
#12484=VERTEX_POINT('',#64533);
#12485=VERTEX_POINT('',#64543);
#12486=VERTEX_POINT('',#64544);
#12487=VERTEX_POINT('',#64546);
#12488=VERTEX_POINT('',#64565);
#12489=VERTEX_POINT('',#64569);
#12490=VERTEX_POINT('',#64570);
#12491=VERTEX_POINT('',#64572);
#12492=VERTEX_POINT('',#64574);
#12493=VERTEX_POINT('',#64593);
#12494=VERTEX_POINT('',#64665);
#12495=VERTEX_POINT('',#64668);
#12496=VERTEX_POINT('',#64670);
#12497=VERTEX_POINT('',#64685);
#12498=VERTEX_POINT('',#64686);
#12499=VERTEX_POINT('',#64691);
#12500=VERTEX_POINT('',#64692);
#12501=VERTEX_POINT('',#64697);
#12502=VERTEX_POINT('',#64699);
#12503=VERTEX_POINT('',#64703);
#12504=VERTEX_POINT('',#64709);
#12505=VERTEX_POINT('',#64717);
#12506=VERTEX_POINT('',#64718);
#12507=VERTEX_POINT('',#64735);
#12508=VERTEX_POINT('',#64737);
#12509=VERTEX_POINT('',#64739);
#12510=VERTEX_POINT('',#64741);
#12511=VERTEX_POINT('',#64743);
#12512=VERTEX_POINT('',#64745);
#12513=VERTEX_POINT('',#64747);
#12514=VERTEX_POINT('',#64750);
#12515=VERTEX_POINT('',#64751);
#12516=VERTEX_POINT('',#64753);
#12517=VERTEX_POINT('',#64755);
#12518=VERTEX_POINT('',#64757);
#12519=VERTEX_POINT('',#64759);
#12520=VERTEX_POINT('',#64761);
#12521=VERTEX_POINT('',#64763);
#12522=VERTEX_POINT('',#64766);
#12523=VERTEX_POINT('',#64767);
#12524=VERTEX_POINT('',#64769);
#12525=VERTEX_POINT('',#64771);
#12526=VERTEX_POINT('',#64773);
#12527=VERTEX_POINT('',#64775);
#12528=VERTEX_POINT('',#64778);
#12529=VERTEX_POINT('',#64779);
#12530=VERTEX_POINT('',#64781);
#12531=VERTEX_POINT('',#64783);
#12532=VERTEX_POINT('',#64785);
#12533=VERTEX_POINT('',#64787);
#12534=VERTEX_POINT('',#64789);
#12535=VERTEX_POINT('',#64791);
#12536=VERTEX_POINT('',#64793);
#12537=VERTEX_POINT('',#64795);
#12538=VERTEX_POINT('',#64797);
#12539=VERTEX_POINT('',#64800);
#12540=VERTEX_POINT('',#64801);
#12541=VERTEX_POINT('',#64803);
#12542=VERTEX_POINT('',#64805);
#12543=VERTEX_POINT('',#64807);
#12544=VERTEX_POINT('',#64809);
#12545=VERTEX_POINT('',#64813);
#12546=VERTEX_POINT('',#64814);
#12547=VERTEX_POINT('',#64816);
#12548=VERTEX_POINT('',#64818);
#12549=VERTEX_POINT('',#64820);
#12550=VERTEX_POINT('',#64822);
#12551=VERTEX_POINT('',#64824);
#12552=VERTEX_POINT('',#64826);
#12553=VERTEX_POINT('',#64846);
#12554=VERTEX_POINT('',#64848);
#12555=VERTEX_POINT('',#64852);
#12556=VERTEX_POINT('',#64856);
#12557=VERTEX_POINT('',#64860);
#12558=VERTEX_POINT('',#64862);
#12559=VERTEX_POINT('',#64866);
#12560=VERTEX_POINT('',#64870);
#12561=VERTEX_POINT('',#64874);
#12562=VERTEX_POINT('',#64878);
#12563=VERTEX_POINT('',#64882);
#12564=VERTEX_POINT('',#64891);
#12565=VERTEX_POINT('',#64892);
#12566=VERTEX_POINT('',#64894);
#12567=VERTEX_POINT('',#64896);
#12568=VERTEX_POINT('',#64898);
#12569=VERTEX_POINT('',#64900);
#12570=VERTEX_POINT('',#64916);
#12571=VERTEX_POINT('',#64918);
#12572=VERTEX_POINT('',#64922);
#12573=VERTEX_POINT('',#64926);
#12574=VERTEX_POINT('',#64930);
#12575=VERTEX_POINT('',#64934);
#12576=VERTEX_POINT('',#64941);
#12577=VERTEX_POINT('',#64943);
#12578=VERTEX_POINT('',#64947);
#12579=VERTEX_POINT('',#64951);
#12580=VERTEX_POINT('',#64955);
#12581=VERTEX_POINT('',#64974);
#12582=VERTEX_POINT('',#64978);
#12583=VERTEX_POINT('',#64980);
#12584=VERTEX_POINT('',#64984);
#12585=VERTEX_POINT('',#64988);
#12586=VERTEX_POINT('',#64992);
#12587=VERTEX_POINT('',#64996);
#12588=VERTEX_POINT('',#65002);
#15733=EDGE_CURVE('',#12411,#12412,#6962,.T.);
#15734=EDGE_CURVE('',#12412,#12413,#10357,.T.);
#15735=EDGE_CURVE('',#12413,#12414,#6963,.T.);
#15736=EDGE_CURVE('',#12414,#12411,#10358,.T.);
#15737=EDGE_CURVE('',#12415,#12416,#10359,.T.);
#15738=EDGE_CURVE('',#12416,#12413,#6964,.T.);
#15739=EDGE_CURVE('',#12412,#12415,#6965,.T.);
#15740=EDGE_CURVE('',#12417,#12418,#10360,.T.);
#15741=EDGE_CURVE('',#12419,#12418,#10361,.T.);
#15742=EDGE_CURVE('',#12419,#12420,#10362,.T.);
#15743=EDGE_CURVE('',#12420,#12417,#10363,.T.);
#15744=EDGE_CURVE('',#12421,#12422,#10364,.T.);
#15745=EDGE_CURVE('',#12423,#12422,#10365,.T.);
#15746=EDGE_CURVE('',#12423,#12424,#10366,.T.);
#15747=EDGE_CURVE('',#12424,#12421,#10367,.T.);
#15748=EDGE_CURVE('',#12425,#12426,#10368,.T.);
#15749=EDGE_CURVE('',#12426,#12421,#6966,.T.);
#15750=EDGE_CURVE('',#12424,#12425,#6967,.T.);
#15751=EDGE_CURVE('',#12427,#12417,#6968,.T.);
#15752=EDGE_CURVE('',#12420,#12428,#6969,.T.);
#15753=EDGE_CURVE('',#12428,#12427,#10369,.T.);
#15754=EDGE_CURVE('',#12429,#12423,#6970,.T.);
#15755=EDGE_CURVE('',#12429,#12425,#10370,.T.);
#15756=EDGE_CURVE('',#12430,#12419,#6971,.T.);
#15757=EDGE_CURVE('',#12430,#12428,#10371,.T.);
#15758=EDGE_CURVE('',#12426,#12431,#10372,.T.);
#15759=EDGE_CURVE('',#12422,#12431,#6972,.T.);
#15760=EDGE_CURVE('',#12427,#12432,#10373,.T.);
#15761=EDGE_CURVE('',#12418,#12432,#6973,.T.);
#15762=EDGE_CURVE('',#12431,#12430,#10374,.T.);
#15763=EDGE_CURVE('',#12432,#12433,#10375,.T.);
#15764=EDGE_CURVE('',#12433,#12416,#6974,.T.);
#15765=EDGE_CURVE('',#12415,#12434,#6975,.T.);
#15766=EDGE_CURVE('',#12434,#12429,#10376,.T.);
#15767=EDGE_CURVE('',#12435,#12436,#374,.T.);
#15768=EDGE_CURVE('',#12436,#12435,#375,.T.);
#15769=EDGE_CURVE('',#12437,#12438,#6976,.T.);
#15770=EDGE_CURVE('',#12438,#12437,#376,.T.);
#15771=EDGE_CURVE('',#12414,#12439,#6977,.T.);
#15772=EDGE_CURVE('',#12440,#12439,#10377,.T.);
#15773=EDGE_CURVE('',#12440,#12411,#6978,.T.);
#15774=EDGE_CURVE('',#12434,#12440,#6979,.T.);
#15775=EDGE_CURVE('',#12439,#12433,#6980,.T.);
#15776=EDGE_CURVE('',#12436,#12441,#6981,.T.);
#15777=EDGE_CURVE('',#12441,#12441,#10378,.T.);
#15778=EDGE_CURVE('',#12437,#12438,#10379,.T.);
#15779=EDGE_CURVE('',#12442,#12442,#10380,.T.);
#15780=EDGE_CURVE('',#12443,#12443,#10381,.T.);
#15781=EDGE_CURVE('',#12443,#12442,#6982,.T.);
#15782=EDGE_CURVE('',#12444,#12444,#10382,.T.);
#15783=EDGE_CURVE('',#12445,#12445,#10383,.T.);
#15784=EDGE_CURVE('',#12445,#12444,#6983,.T.);
#15785=EDGE_CURVE('',#12446,#12447,#10384,.T.);
#15786=EDGE_CURVE('',#12447,#12446,#377,.F.);
#15787=EDGE_CURVE('',#12448,#12449,#6984,.T.);
#15788=EDGE_CURVE('',#12450,#12448,#6985,.T.);
#15789=EDGE_CURVE('',#12451,#12450,#6986,.T.);
#15790=EDGE_CURVE('',#12452,#12451,#6987,.T.);
#15791=EDGE_CURVE('',#12449,#12452,#6988,.T.);
#15792=EDGE_CURVE('',#12453,#12453,#10385,.T.);
#15793=EDGE_CURVE('',#12454,#12455,#378,.F.);
#15794=EDGE_CURVE('',#12455,#12454,#379,.F.);
#15795=EDGE_CURVE('',#12455,#12453,#6989,.T.);
#15796=EDGE_CURVE('',#12456,#12456,#10386,.T.);
#15797=EDGE_CURVE('',#12456,#12457,#6990,.T.);
#15798=EDGE_CURVE('',#12457,#12457,#10387,.T.);
#15799=EDGE_CURVE('',#12458,#12458,#10388,.T.);
#15800=EDGE_CURVE('',#12458,#12459,#6991,.T.);
#15801=EDGE_CURVE('',#12459,#12459,#10389,.T.);
#15802=EDGE_CURVE('',#12446,#12447,#6992,.T.);
#15803=EDGE_CURVE('',#12460,#12461,#6993,.T.);
#15804=EDGE_CURVE('',#12462,#12460,#6994,.T.);
#15805=EDGE_CURVE('',#12463,#12462,#6995,.T.);
#15806=EDGE_CURVE('',#12464,#12463,#6996,.T.);
#15807=EDGE_CURVE('',#12461,#12464,#6997,.T.);
#15808=EDGE_CURVE('',#12464,#12465,#10390,.T.);
#15809=EDGE_CURVE('',#12465,#12466,#6998,.T.);
#15810=EDGE_CURVE('',#12466,#12467,#6999,.T.);
#15811=EDGE_CURVE('',#12467,#12468,#7000,.T.);
#15812=EDGE_CURVE('',#12468,#12450,#10391,.T.);
#15813=EDGE_CURVE('',#12448,#12461,#10392,.T.);
#15814=EDGE_CURVE('',#12449,#12460,#10393,.T.);
#15815=EDGE_CURVE('',#12469,#12462,#10394,.T.);
#15816=EDGE_CURVE('',#12470,#12469,#10395,.T.);
#15817=EDGE_CURVE('',#12471,#12470,#10396,.T.);
#15818=EDGE_CURVE('',#12472,#12471,#10397,.T.);
#15819=EDGE_CURVE('',#12473,#12472,#10398,.T.);
#15820=EDGE_CURVE('',#12474,#12473,#10399,.T.);
#15821=EDGE_CURVE('',#12475,#12474,#10400,.T.);
#15822=EDGE_CURVE('',#12476,#12475,#10401,.T.);
#15823=EDGE_CURVE('',#12452,#12476,#10402,.T.);
#15824=EDGE_CURVE('',#12451,#12477,#10403,.T.);
#15825=EDGE_CURVE('',#12477,#12478,#7001,.T.);
#15826=EDGE_CURVE('',#12478,#12479,#7002,.T.);
#15827=EDGE_CURVE('',#12479,#12480,#7003,.T.);
#15828=EDGE_CURVE('',#12480,#12463,#10404,.T.);
#15829=EDGE_CURVE('',#12481,#12468,#7004,.T.);
#15830=EDGE_CURVE('',#12482,#12481,#380,.T.);
#15831=EDGE_CURVE('',#12477,#12482,#7005,.T.);
#15832=EDGE_CURVE('',#12483,#12480,#7006,.T.);
#15833=EDGE_CURVE('',#12484,#12483,#381,.T.);
#15834=EDGE_CURVE('',#12465,#12484,#7007,.T.);
#15835=EDGE_CURVE('',#12485,#12486,#7008,.T.);
#15836=EDGE_CURVE('',#12486,#12487,#382,.T.);
#15837=EDGE_CURVE('',#12487,#12488,#7009,.T.);
#15838=EDGE_CURVE('',#12488,#12485,#10405,.T.);
#15839=EDGE_CURVE('',#12489,#12490,#10406,.T.);
#15840=EDGE_CURVE('',#12490,#12491,#7010,.T.);
#15841=EDGE_CURVE('',#12492,#12491,#383,.T.);
#15842=EDGE_CURVE('',#12493,#12492,#384,.T.);
#15843=EDGE_CURVE('',#12491,#12493,#385,.T.);
#15844=EDGE_CURVE('',#12490,#12494,#10407,.T.);
#15845=EDGE_CURVE('',#12494,#12484,#7011,.T.);
#15846=EDGE_CURVE('',#12483,#12495,#7012,.T.);
#15847=EDGE_CURVE('',#12495,#12496,#10408,.T.);
#15848=EDGE_CURVE('',#12496,#12482,#7013,.T.);
#15849=EDGE_CURVE('',#12481,#12489,#7014,.T.);
#15850=EDGE_CURVE('',#12494,#12466,#7015,.T.);
#15851=EDGE_CURVE('',#12479,#12495,#7016,.T.);
#15852=EDGE_CURVE('',#12467,#12489,#7017,.T.);
#15853=EDGE_CURVE('',#12496,#12478,#7018,.T.);
#15854=EDGE_CURVE('',#12497,#12498,#10409,.T.);
#15855=EDGE_CURVE('',#12476,#12497,#7019,.T.);
#15856=EDGE_CURVE('',#12498,#12475,#7020,.T.);
#15857=EDGE_CURVE('',#12499,#12500,#10410,.T.);
#15858=EDGE_CURVE('',#12472,#12499,#7021,.T.);
#15859=EDGE_CURVE('',#12500,#12471,#7022,.T.);
#15860=EDGE_CURVE('',#12501,#12469,#7023,.T.);
#15861=EDGE_CURVE('',#12502,#12501,#10411,.T.);
#15862=EDGE_CURVE('',#12470,#12502,#7024,.T.);
#15863=EDGE_CURVE('',#12498,#12503,#10412,.T.);
#15864=EDGE_CURVE('',#12474,#12503,#7025,.T.);
#15865=EDGE_CURVE('',#12500,#12502,#10413,.T.);
#15866=EDGE_CURVE('',#12504,#12473,#7026,.T.);
#15867=EDGE_CURVE('',#12503,#12504,#10414,.T.);
#15868=EDGE_CURVE('',#12499,#12501,#10415,.T.);
#15869=EDGE_CURVE('',#12497,#12504,#10416,.T.);
#15870=EDGE_CURVE('',#12505,#12506,#386,.F.);
#15871=EDGE_CURVE('',#12506,#12507,#10417,.T.);
#15872=EDGE_CURVE('',#12507,#12508,#7027,.T.);
#15873=EDGE_CURVE('',#12508,#12509,#10418,.T.);
#15874=EDGE_CURVE('',#12509,#12510,#7028,.T.);
#15875=EDGE_CURVE('',#12510,#12511,#10419,.T.);
#15876=EDGE_CURVE('',#12511,#12512,#7029,.T.);
#15877=EDGE_CURVE('',#12512,#12513,#10420,.T.);
#15878=EDGE_CURVE('',#12513,#12505,#7030,.T.);
#15879=EDGE_CURVE('',#12514,#12515,#10421,.T.);
#15880=EDGE_CURVE('',#12515,#12516,#7031,.T.);
#15881=EDGE_CURVE('',#12516,#12517,#10422,.T.);
#15882=EDGE_CURVE('',#12517,#12518,#7032,.T.);
#15883=EDGE_CURVE('',#12518,#12519,#10423,.T.);
#15884=EDGE_CURVE('',#12519,#12520,#7033,.T.);
#15885=EDGE_CURVE('',#12520,#12521,#10424,.T.);
#15886=EDGE_CURVE('',#12521,#12514,#7034,.T.);
#15887=EDGE_CURVE('',#12522,#12523,#7035,.T.);
#15888=EDGE_CURVE('',#12523,#12524,#658,.T.);
#15889=EDGE_CURVE('',#12524,#12525,#659,.T.);
#15890=EDGE_CURVE('',#12525,#12526,#7036,.T.);
#15891=EDGE_CURVE('',#12526,#12527,#660,.T.);
#15892=EDGE_CURVE('',#12527,#12522,#661,.T.);
#15893=EDGE_CURVE('',#12528,#12529,#662,.F.);
#15894=EDGE_CURVE('',#12529,#12530,#7037,.T.);
#15895=EDGE_CURVE('',#12530,#12531,#10425,.T.);
#15896=EDGE_CURVE('',#12531,#12532,#10426,.T.);
#15897=EDGE_CURVE('',#12532,#12533,#7038,.T.);
#15898=EDGE_CURVE('',#12533,#12534,#10427,.T.);
#15899=EDGE_CURVE('',#12534,#12535,#7039,.T.);
#15900=EDGE_CURVE('',#12535,#12536,#10428,.T.);
#15901=EDGE_CURVE('',#12536,#12537,#10429,.T.);
#15902=EDGE_CURVE('',#12537,#12538,#7040,.T.);
#15903=EDGE_CURVE('',#12538,#12528,#663,.T.);
#15904=EDGE_CURVE('',#12539,#12540,#664,.T.);
#15905=EDGE_CURVE('',#12540,#12541,#7041,.T.);
#15906=EDGE_CURVE('',#12541,#12542,#665,.T.);
#15907=EDGE_CURVE('',#12542,#12543,#666,.T.);
#15908=EDGE_CURVE('',#12543,#12544,#7042,.T.);
#15909=EDGE_CURVE('',#12544,#12539,#667,.T.);
#15910=EDGE_CURVE('',#12545,#12546,#10430,.T.);
#15911=EDGE_CURVE('',#12546,#12547,#7043,.T.);
#15912=EDGE_CURVE('',#12547,#12548,#10431,.T.);
#15913=EDGE_CURVE('',#12548,#12549,#7044,.T.);
#15914=EDGE_CURVE('',#12549,#12550,#10432,.T.);
#15915=EDGE_CURVE('',#12550,#12551,#7045,.T.);
#15916=EDGE_CURVE('',#12551,#12552,#10433,.T.);
#15917=EDGE_CURVE('',#12552,#12545,#7046,.T.);
#15918=EDGE_CURVE('',#12552,#12516,#7047,.T.);
#15919=EDGE_CURVE('',#12551,#12517,#7048,.T.);
#15920=EDGE_CURVE('',#12545,#12515,#7049,.T.);
#15921=EDGE_CURVE('',#12550,#12518,#7050,.T.);
#15922=EDGE_CURVE('',#12549,#12519,#7051,.T.);
#15923=EDGE_CURVE('',#12548,#12520,#7052,.T.);
#15924=EDGE_CURVE('',#12547,#12521,#7053,.T.);
#15925=EDGE_CURVE('',#12546,#12514,#7054,.T.);
#15926=EDGE_CURVE('',#12553,#12530,#7055,.T.);
#15927=EDGE_CURVE('',#12554,#12553,#668,.T.);
#15928=EDGE_CURVE('',#12554,#12531,#7056,.T.);
#15929=EDGE_CURVE('',#12555,#12529,#7057,.T.);
#15930=EDGE_CURVE('',#12553,#12555,#7058,.T.);
#15931=EDGE_CURVE('',#12556,#12528,#7059,.T.);
#15932=EDGE_CURVE('',#12555,#12556,#669,.F.);
#15933=EDGE_CURVE('',#12557,#12537,#7060,.T.);
#15934=EDGE_CURVE('',#12558,#12557,#7061,.T.);
#15935=EDGE_CURVE('',#12558,#12538,#7062,.T.);
#15936=EDGE_CURVE('',#12559,#12536,#7063,.T.);
#15937=EDGE_CURVE('',#12557,#12559,#10434,.T.);
#15938=EDGE_CURVE('',#12560,#12535,#7064,.T.);
#15939=EDGE_CURVE('',#12559,#12560,#10435,.T.);
#15940=EDGE_CURVE('',#12561,#12534,#7065,.T.);
#15941=EDGE_CURVE('',#12560,#12561,#7066,.T.);
#15942=EDGE_CURVE('',#12562,#12533,#7067,.T.);
#15943=EDGE_CURVE('',#12561,#12562,#10436,.T.);
#15944=EDGE_CURVE('',#12563,#12532,#7068,.T.);
#15945=EDGE_CURVE('',#12562,#12563,#7069,.T.);
#15946=EDGE_CURVE('',#12563,#12554,#10437,.T.);
#15947=EDGE_CURVE('',#12556,#12558,#670,.T.);
#15948=EDGE_CURVE('',#12564,#12565,#671,.T.);
#15949=EDGE_CURVE('',#12565,#12566,#7070,.T.);
#15950=EDGE_CURVE('',#12566,#12567,#672,.T.);
#15951=EDGE_CURVE('',#12567,#12568,#673,.T.);
#15952=EDGE_CURVE('',#12568,#12569,#7071,.T.);
#15953=EDGE_CURVE('',#12569,#12564,#674,.T.);
#15954=EDGE_CURVE('',#12567,#12524,#7072,.T.);
#15955=EDGE_CURVE('',#12566,#12525,#7073,.T.);
#15956=EDGE_CURVE('',#12568,#12523,#7074,.T.);
#15957=EDGE_CURVE('',#12565,#12526,#7075,.T.);
#15958=EDGE_CURVE('',#12564,#12527,#7076,.T.);
#15959=EDGE_CURVE('',#12569,#12522,#7077,.T.);
#15960=EDGE_CURVE('',#12570,#12543,#7078,.T.);
#15961=EDGE_CURVE('',#12571,#12570,#7079,.T.);
#15962=EDGE_CURVE('',#12571,#12544,#7080,.T.);
#15963=EDGE_CURVE('',#12572,#12542,#7081,.T.);
#15964=EDGE_CURVE('',#12570,#12572,#675,.T.);
#15965=EDGE_CURVE('',#12573,#12541,#7082,.T.);
#15966=EDGE_CURVE('',#12572,#12573,#676,.T.);
#15967=EDGE_CURVE('',#12574,#12540,#7083,.T.);
#15968=EDGE_CURVE('',#12573,#12574,#7084,.T.);
#15969=EDGE_CURVE('',#12575,#12571,#677,.T.);
#15970=EDGE_CURVE('',#12575,#12539,#7085,.T.);
#15971=EDGE_CURVE('',#12574,#12575,#678,.T.);
#15972=EDGE_CURVE('',#12576,#12508,#7086,.T.);
#15973=EDGE_CURVE('',#12577,#12576,#10438,.T.);
#15974=EDGE_CURVE('',#12577,#12509,#7087,.T.);
#15975=EDGE_CURVE('',#12578,#12507,#7088,.T.);
#15976=EDGE_CURVE('',#12576,#12578,#7089,.T.);
#15977=EDGE_CURVE('',#12579,#12506,#7090,.T.);
#15978=EDGE_CURVE('',#12578,#12579,#10439,.T.);
#15979=EDGE_CURVE('',#12580,#12505,#7091,.T.);
#15980=EDGE_CURVE('',#12579,#12580,#387,.F.);
#15981=EDGE_CURVE('',#12581,#12513,#7092,.T.);
#15982=EDGE_CURVE('',#12580,#12581,#7093,.T.);
#15983=EDGE_CURVE('',#12582,#12488,#7094,.T.);
#15984=EDGE_CURVE('',#12583,#12582,#10440,.T.);
#15985=EDGE_CURVE('',#12583,#12485,#7095,.T.);
#15986=EDGE_CURVE('',#12584,#12487,#7096,.T.);
#15987=EDGE_CURVE('',#12582,#12584,#7097,.T.);
#15988=EDGE_CURVE('',#12585,#12512,#7098,.T.);
#15989=EDGE_CURVE('',#12581,#12585,#10441,.T.);
#15990=EDGE_CURVE('',#12586,#12511,#7099,.T.);
#15991=EDGE_CURVE('',#12585,#12586,#7100,.T.);
#15992=EDGE_CURVE('',#12587,#12510,#7101,.T.);
#15993=EDGE_CURVE('',#12586,#12587,#10442,.T.);
#15994=EDGE_CURVE('',#12587,#12577,#7102,.T.);
#15995=EDGE_CURVE('',#12588,#12486,#7103,.T.);
#15996=EDGE_CURVE('',#12584,#12588,#388,.T.);
#15997=EDGE_CURVE('',#12588,#12583,#7104,.T.);
#22080=ORIENTED_EDGE('',*,*,#15733,.T.);
#22081=ORIENTED_EDGE('',*,*,#15734,.T.);
#22082=ORIENTED_EDGE('',*,*,#15735,.T.);
#22083=ORIENTED_EDGE('',*,*,#15736,.T.);
#22084=ORIENTED_EDGE('',*,*,#15737,.T.);
#22085=ORIENTED_EDGE('',*,*,#15738,.T.);
#22086=ORIENTED_EDGE('',*,*,#15734,.F.);
#22087=ORIENTED_EDGE('',*,*,#15739,.T.);
#22088=ORIENTED_EDGE('',*,*,#15740,.T.);
#22089=ORIENTED_EDGE('',*,*,#15741,.F.);
#22090=ORIENTED_EDGE('',*,*,#15742,.T.);
#22091=ORIENTED_EDGE('',*,*,#15743,.T.);
#22092=ORIENTED_EDGE('',*,*,#15744,.T.);
#22093=ORIENTED_EDGE('',*,*,#15745,.F.);
#22094=ORIENTED_EDGE('',*,*,#15746,.T.);
#22095=ORIENTED_EDGE('',*,*,#15747,.T.);
#22096=ORIENTED_EDGE('',*,*,#15748,.T.);
#22097=ORIENTED_EDGE('',*,*,#15749,.T.);
#22098=ORIENTED_EDGE('',*,*,#15747,.F.);
#22099=ORIENTED_EDGE('',*,*,#15750,.T.);
#22100=ORIENTED_EDGE('',*,*,#15751,.T.);
#22101=ORIENTED_EDGE('',*,*,#15743,.F.);
#22102=ORIENTED_EDGE('',*,*,#15752,.T.);
#22103=ORIENTED_EDGE('',*,*,#15753,.T.);
#22104=ORIENTED_EDGE('',*,*,#15746,.F.);
#22105=ORIENTED_EDGE('',*,*,#15754,.F.);
#22106=ORIENTED_EDGE('',*,*,#15755,.T.);
#22107=ORIENTED_EDGE('',*,*,#15750,.F.);
#22108=ORIENTED_EDGE('',*,*,#15742,.F.);
#22109=ORIENTED_EDGE('',*,*,#15756,.F.);
#22110=ORIENTED_EDGE('',*,*,#15757,.T.);
#22111=ORIENTED_EDGE('',*,*,#15752,.F.);
#22112=ORIENTED_EDGE('',*,*,#15758,.T.);
#22113=ORIENTED_EDGE('',*,*,#15759,.F.);
#22114=ORIENTED_EDGE('',*,*,#15744,.F.);
#22115=ORIENTED_EDGE('',*,*,#15749,.F.);
#22116=ORIENTED_EDGE('',*,*,#15760,.T.);
#22117=ORIENTED_EDGE('',*,*,#15761,.F.);
#22118=ORIENTED_EDGE('',*,*,#15740,.F.);
#22119=ORIENTED_EDGE('',*,*,#15751,.F.);
#22120=ORIENTED_EDGE('',*,*,#15745,.T.);
#22121=ORIENTED_EDGE('',*,*,#15759,.T.);
#22122=ORIENTED_EDGE('',*,*,#15762,.T.);
#22123=ORIENTED_EDGE('',*,*,#15756,.T.);
#22124=ORIENTED_EDGE('',*,*,#15741,.T.);
#22125=ORIENTED_EDGE('',*,*,#15761,.T.);
#22126=ORIENTED_EDGE('',*,*,#15763,.T.);
#22127=ORIENTED_EDGE('',*,*,#15764,.T.);
#22128=ORIENTED_EDGE('',*,*,#15737,.F.);
#22129=ORIENTED_EDGE('',*,*,#15765,.T.);
#22130=ORIENTED_EDGE('',*,*,#15766,.T.);
#22131=ORIENTED_EDGE('',*,*,#15754,.T.);
#22132=ORIENTED_EDGE('',*,*,#15767,.T.);
#22133=ORIENTED_EDGE('',*,*,#15768,.T.);
#22134=ORIENTED_EDGE('',*,*,#15769,.T.);
#22135=ORIENTED_EDGE('',*,*,#15770,.T.);
#22136=ORIENTED_EDGE('',*,*,#15736,.F.);
#22137=ORIENTED_EDGE('',*,*,#15771,.T.);
#22138=ORIENTED_EDGE('',*,*,#15772,.F.);
#22139=ORIENTED_EDGE('',*,*,#15773,.T.);
#22140=ORIENTED_EDGE('',*,*,#15774,.T.);
#22141=ORIENTED_EDGE('',*,*,#15772,.T.);
#22142=ORIENTED_EDGE('',*,*,#15775,.T.);
#22143=ORIENTED_EDGE('',*,*,#15763,.F.);
#22144=ORIENTED_EDGE('',*,*,#15760,.F.);
#22145=ORIENTED_EDGE('',*,*,#15753,.F.);
#22146=ORIENTED_EDGE('',*,*,#15757,.F.);
#22147=ORIENTED_EDGE('',*,*,#15762,.F.);
#22148=ORIENTED_EDGE('',*,*,#15758,.F.);
#22149=ORIENTED_EDGE('',*,*,#15748,.F.);
#22150=ORIENTED_EDGE('',*,*,#15755,.F.);
#22151=ORIENTED_EDGE('',*,*,#15766,.F.);
#22152=ORIENTED_EDGE('',*,*,#15767,.F.);
#22153=ORIENTED_EDGE('',*,*,#15768,.F.);
#22154=ORIENTED_EDGE('',*,*,#15776,.T.);
#22155=ORIENTED_EDGE('',*,*,#15777,.T.);
#22156=ORIENTED_EDGE('',*,*,#15776,.F.);
#22157=ORIENTED_EDGE('',*,*,#15769,.F.);
#22158=ORIENTED_EDGE('',*,*,#15778,.T.);
#22159=ORIENTED_EDGE('',*,*,#15779,.F.);
#22160=ORIENTED_EDGE('',*,*,#15780,.F.);
#22161=ORIENTED_EDGE('',*,*,#15781,.T.);
#22162=ORIENTED_EDGE('',*,*,#15779,.T.);
#22163=ORIENTED_EDGE('',*,*,#15781,.F.);
#22164=ORIENTED_EDGE('',*,*,#15780,.T.);
#22165=ORIENTED_EDGE('',*,*,#15782,.F.);
#22166=ORIENTED_EDGE('',*,*,#15783,.T.);
#22167=ORIENTED_EDGE('',*,*,#15784,.T.);
#22168=ORIENTED_EDGE('',*,*,#15782,.T.);
#22169=ORIENTED_EDGE('',*,*,#15784,.F.);
#22170=ORIENTED_EDGE('',*,*,#15739,.F.);
#22171=ORIENTED_EDGE('',*,*,#15733,.F.);
#22172=ORIENTED_EDGE('',*,*,#15773,.F.);
#22173=ORIENTED_EDGE('',*,*,#15774,.F.);
#22174=ORIENTED_EDGE('',*,*,#15765,.F.);
#22175=ORIENTED_EDGE('',*,*,#15777,.F.);
#22176=ORIENTED_EDGE('',*,*,#15738,.F.);
#22177=ORIENTED_EDGE('',*,*,#15764,.F.);
#22178=ORIENTED_EDGE('',*,*,#15775,.F.);
#22179=ORIENTED_EDGE('',*,*,#15771,.F.);
#22180=ORIENTED_EDGE('',*,*,#15735,.F.);
#22181=ORIENTED_EDGE('',*,*,#15783,.F.);
#22182=ORIENTED_EDGE('',*,*,#15778,.F.);
#22183=ORIENTED_EDGE('',*,*,#15770,.F.);
#22184=ORIENTED_EDGE('',*,*,#15785,.F.);
#22185=ORIENTED_EDGE('',*,*,#15786,.F.);
#22186=ORIENTED_EDGE('',*,*,#15787,.F.);
#22187=ORIENTED_EDGE('',*,*,#15788,.F.);
#22188=ORIENTED_EDGE('',*,*,#15789,.F.);
#22189=ORIENTED_EDGE('',*,*,#15790,.F.);
#22190=ORIENTED_EDGE('',*,*,#15791,.F.);
#22191=ORIENTED_EDGE('',*,*,#15792,.F.);
#22192=ORIENTED_EDGE('',*,*,#15793,.F.);
#22193=ORIENTED_EDGE('',*,*,#15794,.F.);
#22194=ORIENTED_EDGE('',*,*,#15795,.T.);
#22195=ORIENTED_EDGE('',*,*,#15792,.T.);
#22196=ORIENTED_EDGE('',*,*,#15795,.F.);
#22197=ORIENTED_EDGE('',*,*,#15796,.T.);
#22198=ORIENTED_EDGE('',*,*,#15797,.T.);
#22199=ORIENTED_EDGE('',*,*,#15798,.T.);
#22200=ORIENTED_EDGE('',*,*,#15797,.F.);
#22201=ORIENTED_EDGE('',*,*,#15799,.T.);
#22202=ORIENTED_EDGE('',*,*,#15798,.F.);
#22203=ORIENTED_EDGE('',*,*,#15799,.F.);
#22204=ORIENTED_EDGE('',*,*,#15800,.T.);
#22205=ORIENTED_EDGE('',*,*,#15801,.T.);
#22206=ORIENTED_EDGE('',*,*,#15800,.F.);
#22207=ORIENTED_EDGE('',*,*,#15802,.F.);
#22208=ORIENTED_EDGE('',*,*,#15785,.T.);
#22209=ORIENTED_EDGE('',*,*,#15801,.F.);
#22210=ORIENTED_EDGE('',*,*,#15803,.F.);
#22211=ORIENTED_EDGE('',*,*,#15804,.F.);
#22212=ORIENTED_EDGE('',*,*,#15805,.F.);
#22213=ORIENTED_EDGE('',*,*,#15806,.F.);
#22214=ORIENTED_EDGE('',*,*,#15807,.F.);
#22215=ORIENTED_EDGE('',*,*,#15796,.F.);
#22216=ORIENTED_EDGE('',*,*,#15807,.T.);
#22217=ORIENTED_EDGE('',*,*,#15808,.T.);
#22218=ORIENTED_EDGE('',*,*,#15809,.T.);
#22219=ORIENTED_EDGE('',*,*,#15810,.T.);
#22220=ORIENTED_EDGE('',*,*,#15811,.T.);
#22221=ORIENTED_EDGE('',*,*,#15812,.T.);
#22222=ORIENTED_EDGE('',*,*,#15788,.T.);
#22223=ORIENTED_EDGE('',*,*,#15813,.T.);
#22224=ORIENTED_EDGE('',*,*,#15813,.F.);
#22225=ORIENTED_EDGE('',*,*,#15787,.T.);
#22226=ORIENTED_EDGE('',*,*,#15814,.T.);
#22227=ORIENTED_EDGE('',*,*,#15803,.T.);
#22228=ORIENTED_EDGE('',*,*,#15805,.T.);
#22229=ORIENTED_EDGE('',*,*,#15815,.F.);
#22230=ORIENTED_EDGE('',*,*,#15816,.F.);
#22231=ORIENTED_EDGE('',*,*,#15817,.F.);
#22232=ORIENTED_EDGE('',*,*,#15818,.F.);
#22233=ORIENTED_EDGE('',*,*,#15819,.F.);
#22234=ORIENTED_EDGE('',*,*,#15820,.F.);
#22235=ORIENTED_EDGE('',*,*,#15821,.F.);
#22236=ORIENTED_EDGE('',*,*,#15822,.F.);
#22237=ORIENTED_EDGE('',*,*,#15823,.F.);
#22238=ORIENTED_EDGE('',*,*,#15790,.T.);
#22239=ORIENTED_EDGE('',*,*,#15824,.T.);
#22240=ORIENTED_EDGE('',*,*,#15825,.T.);
#22241=ORIENTED_EDGE('',*,*,#15826,.T.);
#22242=ORIENTED_EDGE('',*,*,#15827,.T.);
#22243=ORIENTED_EDGE('',*,*,#15828,.T.);
#22244=ORIENTED_EDGE('',*,*,#15824,.F.);
#22245=ORIENTED_EDGE('',*,*,#15789,.T.);
#22246=ORIENTED_EDGE('',*,*,#15812,.F.);
#22247=ORIENTED_EDGE('',*,*,#15829,.F.);
#22248=ORIENTED_EDGE('',*,*,#15830,.F.);
#22249=ORIENTED_EDGE('',*,*,#15831,.F.);
#22250=ORIENTED_EDGE('',*,*,#15806,.T.);
#22251=ORIENTED_EDGE('',*,*,#15828,.F.);
#22252=ORIENTED_EDGE('',*,*,#15832,.F.);
#22253=ORIENTED_EDGE('',*,*,#15833,.F.);
#22254=ORIENTED_EDGE('',*,*,#15834,.F.);
#22255=ORIENTED_EDGE('',*,*,#15808,.F.);
#22256=ORIENTED_EDGE('',*,*,#15835,.T.);
#22257=ORIENTED_EDGE('',*,*,#15836,.T.);
#22258=ORIENTED_EDGE('',*,*,#15837,.T.);
#22259=ORIENTED_EDGE('',*,*,#15838,.T.);
#22260=ORIENTED_EDGE('',*,*,#15839,.T.);
#22261=ORIENTED_EDGE('',*,*,#15840,.T.);
#22262=ORIENTED_EDGE('',*,*,#15841,.F.);
#22263=ORIENTED_EDGE('',*,*,#15842,.F.);
#22264=ORIENTED_EDGE('',*,*,#15843,.F.);
#22265=ORIENTED_EDGE('',*,*,#15840,.F.);
#22266=ORIENTED_EDGE('',*,*,#15844,.T.);
#22267=ORIENTED_EDGE('',*,*,#15845,.T.);
#22268=ORIENTED_EDGE('',*,*,#15833,.T.);
#22269=ORIENTED_EDGE('',*,*,#15846,.T.);
#22270=ORIENTED_EDGE('',*,*,#15847,.T.);
#22271=ORIENTED_EDGE('',*,*,#15848,.T.);
#22272=ORIENTED_EDGE('',*,*,#15830,.T.);
#22273=ORIENTED_EDGE('',*,*,#15849,.T.);
#22274=ORIENTED_EDGE('',*,*,#15845,.F.);
#22275=ORIENTED_EDGE('',*,*,#15850,.T.);
#22276=ORIENTED_EDGE('',*,*,#15809,.F.);
#22277=ORIENTED_EDGE('',*,*,#15834,.T.);
#22278=ORIENTED_EDGE('',*,*,#15846,.F.);
#22279=ORIENTED_EDGE('',*,*,#15832,.T.);
#22280=ORIENTED_EDGE('',*,*,#15827,.F.);
#22281=ORIENTED_EDGE('',*,*,#15851,.T.);
#22282=ORIENTED_EDGE('',*,*,#15839,.F.);
#22283=ORIENTED_EDGE('',*,*,#15852,.F.);
#22284=ORIENTED_EDGE('',*,*,#15810,.F.);
#22285=ORIENTED_EDGE('',*,*,#15850,.F.);
#22286=ORIENTED_EDGE('',*,*,#15844,.F.);
#22287=ORIENTED_EDGE('',*,*,#15847,.F.);
#22288=ORIENTED_EDGE('',*,*,#15851,.F.);
#22289=ORIENTED_EDGE('',*,*,#15826,.F.);
#22290=ORIENTED_EDGE('',*,*,#15853,.F.);
#22291=ORIENTED_EDGE('',*,*,#15849,.F.);
#22292=ORIENTED_EDGE('',*,*,#15829,.T.);
#22293=ORIENTED_EDGE('',*,*,#15811,.F.);
#22294=ORIENTED_EDGE('',*,*,#15852,.T.);
#22295=ORIENTED_EDGE('',*,*,#15848,.F.);
#22296=ORIENTED_EDGE('',*,*,#15853,.T.);
#22297=ORIENTED_EDGE('',*,*,#15825,.F.);
#22298=ORIENTED_EDGE('',*,*,#15831,.T.);
#22299=ORIENTED_EDGE('',*,*,#15854,.F.);
#22300=ORIENTED_EDGE('',*,*,#15855,.F.);
#22301=ORIENTED_EDGE('',*,*,#15822,.T.);
#22302=ORIENTED_EDGE('',*,*,#15856,.F.);
#22303=ORIENTED_EDGE('',*,*,#15857,.F.);
#22304=ORIENTED_EDGE('',*,*,#15858,.F.);
#22305=ORIENTED_EDGE('',*,*,#15818,.T.);
#22306=ORIENTED_EDGE('',*,*,#15859,.F.);
#22307=ORIENTED_EDGE('',*,*,#15816,.T.);
#22308=ORIENTED_EDGE('',*,*,#15860,.F.);
#22309=ORIENTED_EDGE('',*,*,#15861,.F.);
#22310=ORIENTED_EDGE('',*,*,#15862,.F.);
#22311=ORIENTED_EDGE('',*,*,#15863,.F.);
#22312=ORIENTED_EDGE('',*,*,#15856,.T.);
#22313=ORIENTED_EDGE('',*,*,#15821,.T.);
#22314=ORIENTED_EDGE('',*,*,#15864,.T.);
#22315=ORIENTED_EDGE('',*,*,#15862,.T.);
#22316=ORIENTED_EDGE('',*,*,#15865,.F.);
#22317=ORIENTED_EDGE('',*,*,#15859,.T.);
#22318=ORIENTED_EDGE('',*,*,#15817,.T.);
#22319=ORIENTED_EDGE('',*,*,#15820,.T.);
#22320=ORIENTED_EDGE('',*,*,#15866,.F.);
#22321=ORIENTED_EDGE('',*,*,#15867,.F.);
#22322=ORIENTED_EDGE('',*,*,#15864,.F.);
#22323=ORIENTED_EDGE('',*,*,#15857,.T.);
#22324=ORIENTED_EDGE('',*,*,#15865,.T.);
#22325=ORIENTED_EDGE('',*,*,#15861,.T.);
#22326=ORIENTED_EDGE('',*,*,#15868,.F.);
#22327=ORIENTED_EDGE('',*,*,#15854,.T.);
#22328=ORIENTED_EDGE('',*,*,#15863,.T.);
#22329=ORIENTED_EDGE('',*,*,#15867,.T.);
#22330=ORIENTED_EDGE('',*,*,#15869,.F.);
#22331=ORIENTED_EDGE('',*,*,#15814,.F.);
#22332=ORIENTED_EDGE('',*,*,#15791,.T.);
#22333=ORIENTED_EDGE('',*,*,#15823,.T.);
#22334=ORIENTED_EDGE('',*,*,#15855,.T.);
#22335=ORIENTED_EDGE('',*,*,#15869,.T.);
#22336=ORIENTED_EDGE('',*,*,#15866,.T.);
#22337=ORIENTED_EDGE('',*,*,#15819,.T.);
#22338=ORIENTED_EDGE('',*,*,#15858,.T.);
#22339=ORIENTED_EDGE('',*,*,#15868,.T.);
#22340=ORIENTED_EDGE('',*,*,#15860,.T.);
#22341=ORIENTED_EDGE('',*,*,#15815,.T.);
#22342=ORIENTED_EDGE('',*,*,#15804,.T.);
#22343=ORIENTED_EDGE('',*,*,#15793,.T.);
#22344=ORIENTED_EDGE('',*,*,#15794,.T.);
#22345=ORIENTED_EDGE('',*,*,#15870,.T.);
#22346=ORIENTED_EDGE('',*,*,#15871,.T.);
#22347=ORIENTED_EDGE('',*,*,#15872,.T.);
#22348=ORIENTED_EDGE('',*,*,#15873,.T.);
#22349=ORIENTED_EDGE('',*,*,#15874,.T.);
#22350=ORIENTED_EDGE('',*,*,#15875,.T.);
#22351=ORIENTED_EDGE('',*,*,#15876,.T.);
#22352=ORIENTED_EDGE('',*,*,#15877,.T.);
#22353=ORIENTED_EDGE('',*,*,#15878,.T.);
#22354=ORIENTED_EDGE('',*,*,#15879,.T.);
#22355=ORIENTED_EDGE('',*,*,#15880,.T.);
#22356=ORIENTED_EDGE('',*,*,#15881,.T.);
#22357=ORIENTED_EDGE('',*,*,#15882,.T.);
#22358=ORIENTED_EDGE('',*,*,#15883,.T.);
#22359=ORIENTED_EDGE('',*,*,#15884,.T.);
#22360=ORIENTED_EDGE('',*,*,#15885,.T.);
#22361=ORIENTED_EDGE('',*,*,#15886,.T.);
#22362=ORIENTED_EDGE('',*,*,#15841,.T.);
#22363=ORIENTED_EDGE('',*,*,#15843,.T.);
#22364=ORIENTED_EDGE('',*,*,#15842,.T.);
#22365=ORIENTED_EDGE('',*,*,#15802,.T.);
#22366=ORIENTED_EDGE('',*,*,#15786,.T.);
#22367=ORIENTED_EDGE('',*,*,#15887,.T.);
#22368=ORIENTED_EDGE('',*,*,#15888,.T.);
#22369=ORIENTED_EDGE('',*,*,#15889,.T.);
#22370=ORIENTED_EDGE('',*,*,#15890,.T.);
#22371=ORIENTED_EDGE('',*,*,#15891,.T.);
#22372=ORIENTED_EDGE('',*,*,#15892,.T.);
#22373=ORIENTED_EDGE('',*,*,#15893,.T.);
#22374=ORIENTED_EDGE('',*,*,#15894,.T.);
#22375=ORIENTED_EDGE('',*,*,#15895,.T.);
#22376=ORIENTED_EDGE('',*,*,#15896,.T.);
#22377=ORIENTED_EDGE('',*,*,#15897,.T.);
#22378=ORIENTED_EDGE('',*,*,#15898,.T.);
#22379=ORIENTED_EDGE('',*,*,#15899,.T.);
#22380=ORIENTED_EDGE('',*,*,#15900,.T.);
#22381=ORIENTED_EDGE('',*,*,#15901,.T.);
#22382=ORIENTED_EDGE('',*,*,#15902,.T.);
#22383=ORIENTED_EDGE('',*,*,#15903,.T.);
#22384=ORIENTED_EDGE('',*,*,#15904,.T.);
#22385=ORIENTED_EDGE('',*,*,#15905,.T.);
#22386=ORIENTED_EDGE('',*,*,#15906,.T.);
#22387=ORIENTED_EDGE('',*,*,#15907,.T.);
#22388=ORIENTED_EDGE('',*,*,#15908,.T.);
#22389=ORIENTED_EDGE('',*,*,#15909,.T.);
#22390=ORIENTED_EDGE('',*,*,#15910,.T.);
#22391=ORIENTED_EDGE('',*,*,#15911,.T.);
#22392=ORIENTED_EDGE('',*,*,#15912,.T.);
#22393=ORIENTED_EDGE('',*,*,#15913,.T.);
#22394=ORIENTED_EDGE('',*,*,#15914,.T.);
#22395=ORIENTED_EDGE('',*,*,#15915,.T.);
#22396=ORIENTED_EDGE('',*,*,#15916,.T.);
#22397=ORIENTED_EDGE('',*,*,#15917,.T.);
#22398=ORIENTED_EDGE('',*,*,#15881,.F.);
#22399=ORIENTED_EDGE('',*,*,#15918,.F.);
#22400=ORIENTED_EDGE('',*,*,#15916,.F.);
#22401=ORIENTED_EDGE('',*,*,#15919,.T.);
#22402=ORIENTED_EDGE('',*,*,#15880,.F.);
#22403=ORIENTED_EDGE('',*,*,#15920,.F.);
#22404=ORIENTED_EDGE('',*,*,#15917,.F.);
#22405=ORIENTED_EDGE('',*,*,#15918,.T.);
#22406=ORIENTED_EDGE('',*,*,#15882,.F.);
#22407=ORIENTED_EDGE('',*,*,#15919,.F.);
#22408=ORIENTED_EDGE('',*,*,#15915,.F.);
#22409=ORIENTED_EDGE('',*,*,#15921,.T.);
#22410=ORIENTED_EDGE('',*,*,#15883,.F.);
#22411=ORIENTED_EDGE('',*,*,#15921,.F.);
#22412=ORIENTED_EDGE('',*,*,#15914,.F.);
#22413=ORIENTED_EDGE('',*,*,#15922,.T.);
#22414=ORIENTED_EDGE('',*,*,#15884,.F.);
#22415=ORIENTED_EDGE('',*,*,#15922,.F.);
#22416=ORIENTED_EDGE('',*,*,#15913,.F.);
#22417=ORIENTED_EDGE('',*,*,#15923,.T.);
#22418=ORIENTED_EDGE('',*,*,#15885,.F.);
#22419=ORIENTED_EDGE('',*,*,#15923,.F.);
#22420=ORIENTED_EDGE('',*,*,#15912,.F.);
#22421=ORIENTED_EDGE('',*,*,#15924,.T.);
#22422=ORIENTED_EDGE('',*,*,#15886,.F.);
#22423=ORIENTED_EDGE('',*,*,#15924,.F.);
#22424=ORIENTED_EDGE('',*,*,#15911,.F.);
#22425=ORIENTED_EDGE('',*,*,#15925,.T.);
#22426=ORIENTED_EDGE('',*,*,#15879,.F.);
#22427=ORIENTED_EDGE('',*,*,#15925,.F.);
#22428=ORIENTED_EDGE('',*,*,#15910,.F.);
#22429=ORIENTED_EDGE('',*,*,#15920,.T.);
#22430=ORIENTED_EDGE('',*,*,#15895,.F.);
#22431=ORIENTED_EDGE('',*,*,#15926,.F.);
#22432=ORIENTED_EDGE('',*,*,#15927,.F.);
#22433=ORIENTED_EDGE('',*,*,#15928,.T.);
#22434=ORIENTED_EDGE('',*,*,#15894,.F.);
#22435=ORIENTED_EDGE('',*,*,#15929,.F.);
#22436=ORIENTED_EDGE('',*,*,#15930,.F.);
#22437=ORIENTED_EDGE('',*,*,#15926,.T.);
#22438=ORIENTED_EDGE('',*,*,#15893,.F.);
#22439=ORIENTED_EDGE('',*,*,#15931,.F.);
#22440=ORIENTED_EDGE('',*,*,#15932,.F.);
#22441=ORIENTED_EDGE('',*,*,#15929,.T.);
#22442=ORIENTED_EDGE('',*,*,#15902,.F.);
#22443=ORIENTED_EDGE('',*,*,#15933,.F.);
#22444=ORIENTED_EDGE('',*,*,#15934,.F.);
#22445=ORIENTED_EDGE('',*,*,#15935,.T.);
#22446=ORIENTED_EDGE('',*,*,#15901,.F.);
#22447=ORIENTED_EDGE('',*,*,#15936,.F.);
#22448=ORIENTED_EDGE('',*,*,#15937,.F.);
#22449=ORIENTED_EDGE('',*,*,#15933,.T.);
#22450=ORIENTED_EDGE('',*,*,#15900,.F.);
#22451=ORIENTED_EDGE('',*,*,#15938,.F.);
#22452=ORIENTED_EDGE('',*,*,#15939,.F.);
#22453=ORIENTED_EDGE('',*,*,#15936,.T.);
#22454=ORIENTED_EDGE('',*,*,#15899,.F.);
#22455=ORIENTED_EDGE('',*,*,#15940,.F.);
#22456=ORIENTED_EDGE('',*,*,#15941,.F.);
#22457=ORIENTED_EDGE('',*,*,#15938,.T.);
#22458=ORIENTED_EDGE('',*,*,#15898,.F.);
#22459=ORIENTED_EDGE('',*,*,#15942,.F.);
#22460=ORIENTED_EDGE('',*,*,#15943,.F.);
#22461=ORIENTED_EDGE('',*,*,#15940,.T.);
#22462=ORIENTED_EDGE('',*,*,#15897,.F.);
#22463=ORIENTED_EDGE('',*,*,#15944,.F.);
#22464=ORIENTED_EDGE('',*,*,#15945,.F.);
#22465=ORIENTED_EDGE('',*,*,#15942,.T.);
#22466=ORIENTED_EDGE('',*,*,#15896,.F.);
#22467=ORIENTED_EDGE('',*,*,#15928,.F.);
#22468=ORIENTED_EDGE('',*,*,#15946,.F.);
#22469=ORIENTED_EDGE('',*,*,#15944,.T.);
#22470=ORIENTED_EDGE('',*,*,#15903,.F.);
#22471=ORIENTED_EDGE('',*,*,#15935,.F.);
#22472=ORIENTED_EDGE('',*,*,#15947,.F.);
#22473=ORIENTED_EDGE('',*,*,#15931,.T.);
#22474=ORIENTED_EDGE('',*,*,#15932,.T.);
#22475=ORIENTED_EDGE('',*,*,#15947,.T.);
#22476=ORIENTED_EDGE('',*,*,#15934,.T.);
#22477=ORIENTED_EDGE('',*,*,#15937,.T.);
#22478=ORIENTED_EDGE('',*,*,#15939,.T.);
#22479=ORIENTED_EDGE('',*,*,#15941,.T.);
#22480=ORIENTED_EDGE('',*,*,#15943,.T.);
#22481=ORIENTED_EDGE('',*,*,#15945,.T.);
#22482=ORIENTED_EDGE('',*,*,#15946,.T.);
#22483=ORIENTED_EDGE('',*,*,#15927,.T.);
#22484=ORIENTED_EDGE('',*,*,#15930,.T.);
#22485=ORIENTED_EDGE('',*,*,#15948,.T.);
#22486=ORIENTED_EDGE('',*,*,#15949,.T.);
#22487=ORIENTED_EDGE('',*,*,#15950,.T.);
#22488=ORIENTED_EDGE('',*,*,#15951,.T.);
#22489=ORIENTED_EDGE('',*,*,#15952,.T.);
#22490=ORIENTED_EDGE('',*,*,#15953,.T.);
#22491=ORIENTED_EDGE('',*,*,#15889,.F.);
#22492=ORIENTED_EDGE('',*,*,#15954,.F.);
#22493=ORIENTED_EDGE('',*,*,#15950,.F.);
#22494=ORIENTED_EDGE('',*,*,#15955,.T.);
#22495=ORIENTED_EDGE('',*,*,#15888,.F.);
#22496=ORIENTED_EDGE('',*,*,#15956,.F.);
#22497=ORIENTED_EDGE('',*,*,#15951,.F.);
#22498=ORIENTED_EDGE('',*,*,#15954,.T.);
#22499=ORIENTED_EDGE('',*,*,#15890,.F.);
#22500=ORIENTED_EDGE('',*,*,#15955,.F.);
#22501=ORIENTED_EDGE('',*,*,#15949,.F.);
#22502=ORIENTED_EDGE('',*,*,#15957,.T.);
#22503=ORIENTED_EDGE('',*,*,#15891,.F.);
#22504=ORIENTED_EDGE('',*,*,#15957,.F.);
#22505=ORIENTED_EDGE('',*,*,#15948,.F.);
#22506=ORIENTED_EDGE('',*,*,#15958,.T.);
#22507=ORIENTED_EDGE('',*,*,#15892,.F.);
#22508=ORIENTED_EDGE('',*,*,#15958,.F.);
#22509=ORIENTED_EDGE('',*,*,#15953,.F.);
#22510=ORIENTED_EDGE('',*,*,#15959,.T.);
#22511=ORIENTED_EDGE('',*,*,#15887,.F.);
#22512=ORIENTED_EDGE('',*,*,#15959,.F.);
#22513=ORIENTED_EDGE('',*,*,#15952,.F.);
#22514=ORIENTED_EDGE('',*,*,#15956,.T.);
#22515=ORIENTED_EDGE('',*,*,#15908,.F.);
#22516=ORIENTED_EDGE('',*,*,#15960,.F.);
#22517=ORIENTED_EDGE('',*,*,#15961,.F.);
#22518=ORIENTED_EDGE('',*,*,#15962,.T.);
#22519=ORIENTED_EDGE('',*,*,#15907,.F.);
#22520=ORIENTED_EDGE('',*,*,#15963,.F.);
#22521=ORIENTED_EDGE('',*,*,#15964,.F.);
#22522=ORIENTED_EDGE('',*,*,#15960,.T.);
#22523=ORIENTED_EDGE('',*,*,#15906,.F.);
#22524=ORIENTED_EDGE('',*,*,#15965,.F.);
#22525=ORIENTED_EDGE('',*,*,#15966,.F.);
#22526=ORIENTED_EDGE('',*,*,#15963,.T.);
#22527=ORIENTED_EDGE('',*,*,#15905,.F.);
#22528=ORIENTED_EDGE('',*,*,#15967,.F.);
#22529=ORIENTED_EDGE('',*,*,#15968,.F.);
#22530=ORIENTED_EDGE('',*,*,#15965,.T.);
#22531=ORIENTED_EDGE('',*,*,#15909,.F.);
#22532=ORIENTED_EDGE('',*,*,#15962,.F.);
#22533=ORIENTED_EDGE('',*,*,#15969,.F.);
#22534=ORIENTED_EDGE('',*,*,#15970,.T.);
#22535=ORIENTED_EDGE('',*,*,#15904,.F.);
#22536=ORIENTED_EDGE('',*,*,#15970,.F.);
#22537=ORIENTED_EDGE('',*,*,#15971,.F.);
#22538=ORIENTED_EDGE('',*,*,#15967,.T.);
#22539=ORIENTED_EDGE('',*,*,#15966,.T.);
#22540=ORIENTED_EDGE('',*,*,#15968,.T.);
#22541=ORIENTED_EDGE('',*,*,#15971,.T.);
#22542=ORIENTED_EDGE('',*,*,#15969,.T.);
#22543=ORIENTED_EDGE('',*,*,#15961,.T.);
#22544=ORIENTED_EDGE('',*,*,#15964,.T.);
#22545=ORIENTED_EDGE('',*,*,#15873,.F.);
#22546=ORIENTED_EDGE('',*,*,#15972,.F.);
#22547=ORIENTED_EDGE('',*,*,#15973,.F.);
#22548=ORIENTED_EDGE('',*,*,#15974,.T.);
#22549=ORIENTED_EDGE('',*,*,#15872,.F.);
#22550=ORIENTED_EDGE('',*,*,#15975,.F.);
#22551=ORIENTED_EDGE('',*,*,#15976,.F.);
#22552=ORIENTED_EDGE('',*,*,#15972,.T.);
#22553=ORIENTED_EDGE('',*,*,#15871,.F.);
#22554=ORIENTED_EDGE('',*,*,#15977,.F.);
#22555=ORIENTED_EDGE('',*,*,#15978,.F.);
#22556=ORIENTED_EDGE('',*,*,#15975,.T.);
#22557=ORIENTED_EDGE('',*,*,#15870,.F.);
#22558=ORIENTED_EDGE('',*,*,#15979,.F.);
#22559=ORIENTED_EDGE('',*,*,#15980,.F.);
#22560=ORIENTED_EDGE('',*,*,#15977,.T.);
#22561=ORIENTED_EDGE('',*,*,#15878,.F.);
#22562=ORIENTED_EDGE('',*,*,#15981,.F.);
#22563=ORIENTED_EDGE('',*,*,#15982,.F.);
#22564=ORIENTED_EDGE('',*,*,#15979,.T.);
#22565=ORIENTED_EDGE('',*,*,#15838,.F.);
#22566=ORIENTED_EDGE('',*,*,#15983,.F.);
#22567=ORIENTED_EDGE('',*,*,#15984,.F.);
#22568=ORIENTED_EDGE('',*,*,#15985,.T.);
#22569=ORIENTED_EDGE('',*,*,#15837,.F.);
#22570=ORIENTED_EDGE('',*,*,#15986,.F.);
#22571=ORIENTED_EDGE('',*,*,#15987,.F.);
#22572=ORIENTED_EDGE('',*,*,#15983,.T.);
#22573=ORIENTED_EDGE('',*,*,#15877,.F.);
#22574=ORIENTED_EDGE('',*,*,#15988,.F.);
#22575=ORIENTED_EDGE('',*,*,#15989,.F.);
#22576=ORIENTED_EDGE('',*,*,#15981,.T.);
#22577=ORIENTED_EDGE('',*,*,#15876,.F.);
#22578=ORIENTED_EDGE('',*,*,#15990,.F.);
#22579=ORIENTED_EDGE('',*,*,#15991,.F.);
#22580=ORIENTED_EDGE('',*,*,#15988,.T.);
#22581=ORIENTED_EDGE('',*,*,#15875,.F.);
#22582=ORIENTED_EDGE('',*,*,#15992,.F.);
#22583=ORIENTED_EDGE('',*,*,#15993,.F.);
#22584=ORIENTED_EDGE('',*,*,#15990,.T.);
#22585=ORIENTED_EDGE('',*,*,#15874,.F.);
#22586=ORIENTED_EDGE('',*,*,#15974,.F.);
#22587=ORIENTED_EDGE('',*,*,#15994,.F.);
#22588=ORIENTED_EDGE('',*,*,#15992,.T.);
#22589=ORIENTED_EDGE('',*,*,#15836,.F.);
#22590=ORIENTED_EDGE('',*,*,#15995,.F.);
#22591=ORIENTED_EDGE('',*,*,#15996,.F.);
#22592=ORIENTED_EDGE('',*,*,#15986,.T.);
#22593=ORIENTED_EDGE('',*,*,#15835,.F.);
#22594=ORIENTED_EDGE('',*,*,#15985,.F.);
#22595=ORIENTED_EDGE('',*,*,#15997,.F.);
#22596=ORIENTED_EDGE('',*,*,#15995,.T.);
#22597=ORIENTED_EDGE('',*,*,#15980,.T.);
#22598=ORIENTED_EDGE('',*,*,#15982,.T.);
#22599=ORIENTED_EDGE('',*,*,#15989,.T.);
#22600=ORIENTED_EDGE('',*,*,#15991,.T.);
#22601=ORIENTED_EDGE('',*,*,#15993,.T.);
#22602=ORIENTED_EDGE('',*,*,#15994,.T.);
#22603=ORIENTED_EDGE('',*,*,#15973,.T.);
#22604=ORIENTED_EDGE('',*,*,#15976,.T.);
#22605=ORIENTED_EDGE('',*,*,#15978,.T.);
#22606=ORIENTED_EDGE('',*,*,#15987,.T.);
#22607=ORIENTED_EDGE('',*,*,#15996,.T.);
#22608=ORIENTED_EDGE('',*,*,#15997,.T.);
#22609=ORIENTED_EDGE('',*,*,#15984,.T.);
#24109=CYLINDRICAL_SURFACE('',#28017,17.5);
#24110=CYLINDRICAL_SURFACE('',#28019,17.5);
#24111=CYLINDRICAL_SURFACE('',#28021,13.);
#24112=CYLINDRICAL_SURFACE('',#28023,13.);
#24113=CYLINDRICAL_SURFACE('',#28025,13.);
#24114=CYLINDRICAL_SURFACE('',#28027,13.);
#24115=CYLINDRICAL_SURFACE('',#28029,27.5);
#24116=CYLINDRICAL_SURFACE('',#28033,6.00000000000001);
#24117=CYLINDRICAL_SURFACE('',#28036,2.5);
#24118=CYLINDRICAL_SURFACE('',#28041,3.3);
#24119=CYLINDRICAL_SURFACE('',#28045,2.5);
#24120=CYLINDRICAL_SURFACE('',#28049,5.5);
#24121=CYLINDRICAL_SURFACE('',#28050,5.5);
#24122=CYLINDRICAL_SURFACE('',#28054,2.5);
#24123=CYLINDRICAL_SURFACE('',#28055,2.5);
#24124=CYLINDRICAL_SURFACE('',#28060,3.3);
#24125=CYLINDRICAL_SURFACE('',#28082,6.);
#24126=CYLINDRICAL_SURFACE('',#28083,6.);
#24127=CYLINDRICAL_SURFACE('',#28084,27.5);
#24128=CYLINDRICAL_SURFACE('',#28086,2.1);
#24129=CYLINDRICAL_SURFACE('',#28096,13.);
#24130=CYLINDRICAL_SURFACE('',#28098,13.);
#24131=CYLINDRICAL_SURFACE('',#28100,13.);
#24132=CYLINDRICAL_SURFACE('',#28102,17.5);
#24133=CYLINDRICAL_SURFACE('',#28104,17.5);
#24134=CYLINDRICAL_SURFACE('',#28106,13.);
#24135=CYLINDRICAL_SURFACE('',#28112,27.5);
#24136=CYLINDRICAL_SURFACE('',#28136,27.);
#24137=CYLINDRICAL_SURFACE('',#28167,27.);
#24138=CYLINDRICAL_SURFACE('',#28168,27.);
#24139=CYLINDRICAL_SURFACE('',#28189,27.);
#24140=CYLINDRICAL_SURFACE('',#28195,1.4361111111);
#24141=CYLINDRICAL_SURFACE('',#28206,0.4033333333);
#24142=CYLINDRICAL_SURFACE('',#28208,27.);
#25306=ADVANCED_FACE('',(#3353),#2055,.T.);
#25307=ADVANCED_FACE('',(#3354),#553,.T.);
#25308=ADVANCED_FACE('',(#3355),#2056,.T.);
#25309=ADVANCED_FACE('',(#3356),#2057,.T.);
#25310=ADVANCED_FACE('',(#3357),#24109,.F.);
#25311=ADVANCED_FACE('',(#3358),#24110,.F.);
#25312=ADVANCED_FACE('',(#3359),#24111,.F.);
#25313=ADVANCED_FACE('',(#3360),#24112,.F.);
#25314=ADVANCED_FACE('',(#3361),#24113,.F.);
#25315=ADVANCED_FACE('',(#3362),#24114,.F.);
#25316=ADVANCED_FACE('',(#3363,#1408,#1409),#24115,.T.);
#25317=ADVANCED_FACE('',(#3364),#24116,.F.);
#25318=ADVANCED_FACE('',(#3365),#2058,.F.);
#25319=ADVANCED_FACE('',(#3366),#24117,.F.);
#25320=ADVANCED_FACE('',(#3367,#1410),#2059,.F.);
#25321=ADVANCED_FACE('',(#3368),#24118,.F.);
#25322=ADVANCED_FACE('',(#3369,#1411),#2060,.F.);
#25323=ADVANCED_FACE('',(#3370),#24119,.F.);
#25324=ADVANCED_FACE('',(#3371,#1412),#2061,.T.);
#25325=ADVANCED_FACE('',(#3372,#1413),#2062,.T.);
#25326=ADVANCED_FACE('',(#3373),#24120,.F.);
#25327=ADVANCED_FACE('',(#3374),#24121,.F.);
#25328=ADVANCED_FACE('',(#3375,#1414),#2063,.T.);
#25329=ADVANCED_FACE('',(#3376),#24122,.F.);
#25330=ADVANCED_FACE('',(#3377),#24123,.F.);
#25331=ADVANCED_FACE('',(#3378,#1415),#2064,.F.);
#25332=ADVANCED_FACE('',(#3379),#24124,.F.);
#25333=ADVANCED_FACE('',(#3380,#1416),#2065,.F.);
#25334=ADVANCED_FACE('',(#3381,#1417),#2066,.T.);
#25335=ADVANCED_FACE('',(#3382),#2067,.T.);
#25336=ADVANCED_FACE('',(#3383),#554,.T.);
#25337=ADVANCED_FACE('',(#3384),#2068,.F.);
#25338=ADVANCED_FACE('',(#3385),#24125,.F.);
#25339=ADVANCED_FACE('',(#3386),#24126,.F.);
#25340=ADVANCED_FACE('',(#3387),#24127,.T.);
#25341=ADVANCED_FACE('',(#3388),#24128,.F.);
#25342=ADVANCED_FACE('',(#3389),#2069,.T.);
#25343=ADVANCED_FACE('',(#3390),#2070,.T.);
#25344=ADVANCED_FACE('',(#3391),#2071,.F.);
#25345=ADVANCED_FACE('',(#3392),#2072,.F.);
#25346=ADVANCED_FACE('',(#3393),#2073,.T.);
#25347=ADVANCED_FACE('',(#3394),#2074,.T.);
#25348=ADVANCED_FACE('',(#3395),#24129,.F.);
#25349=ADVANCED_FACE('',(#3396),#24130,.F.);
#25350=ADVANCED_FACE('',(#3397),#24131,.F.);
#25351=ADVANCED_FACE('',(#3398),#24132,.F.);
#25352=ADVANCED_FACE('',(#3399),#24133,.F.);
#25353=ADVANCED_FACE('',(#3400),#24134,.F.);
#25354=ADVANCED_FACE('',(#3401),#2075,.T.);
#25355=ADVANCED_FACE('',(#3402),#2076,.T.);
#25356=ADVANCED_FACE('',(#3403,#1418,#1419,#1420,#1421,#1422,#1423,#1424,
#1425),#24135,.T.);
#25357=ADVANCED_FACE('',(#3404),#24136,.T.);
#25358=ADVANCED_FACE('',(#3405),#2077,.F.);
#25359=ADVANCED_FACE('',(#3406),#2078,.F.);
#25360=ADVANCED_FACE('',(#3407),#2079,.F.);
#25361=ADVANCED_FACE('',(#3408),#2080,.F.);
#25362=ADVANCED_FACE('',(#3409),#2081,.F.);
#25363=ADVANCED_FACE('',(#3410),#2082,.F.);
#25364=ADVANCED_FACE('',(#3411),#2083,.F.);
#25365=ADVANCED_FACE('',(#3412),#2084,.F.);
#25366=ADVANCED_FACE('',(#3413),#2085,.F.);
#25367=ADVANCED_FACE('',(#3414),#2086,.F.);
#25368=ADVANCED_FACE('',(#3415),#2087,.F.);
#25369=ADVANCED_FACE('',(#3416),#2088,.F.);
#25370=ADVANCED_FACE('',(#3417),#2089,.F.);
#25371=ADVANCED_FACE('',(#3418),#2090,.F.);
#25372=ADVANCED_FACE('',(#3419),#2091,.F.);
#25373=ADVANCED_FACE('',(#3420),#2092,.F.);
#25374=ADVANCED_FACE('',(#3421),#2093,.F.);
#25375=ADVANCED_FACE('',(#3422),#2094,.F.);
#25376=ADVANCED_FACE('',(#3423),#2095,.F.);
#25377=ADVANCED_FACE('',(#3424),#24137,.T.);
#25378=ADVANCED_FACE('',(#3425),#24138,.T.);
#25379=ADVANCED_FACE('',(#3426),#2096,.F.);
#25380=ADVANCED_FACE('',(#3427),#2097,.F.);
#25381=ADVANCED_FACE('',(#3428),#2098,.F.);
#25382=ADVANCED_FACE('',(#3429),#2099,.F.);
#25383=ADVANCED_FACE('',(#3430),#2100,.F.);
#25384=ADVANCED_FACE('',(#3431),#2101,.F.);
#25385=ADVANCED_FACE('',(#3432),#2102,.F.);
#25386=ADVANCED_FACE('',(#3433),#2103,.F.);
#25387=ADVANCED_FACE('',(#3434),#2104,.F.);
#25388=ADVANCED_FACE('',(#3435),#2105,.F.);
#25389=ADVANCED_FACE('',(#3436),#2106,.F.);
#25390=ADVANCED_FACE('',(#3437),#2107,.F.);
#25391=ADVANCED_FACE('',(#3438),#24139,.T.);
#25392=ADVANCED_FACE('',(#3439),#2108,.F.);
#25393=ADVANCED_FACE('',(#3440),#2109,.F.);
#25394=ADVANCED_FACE('',(#3441),#2110,.F.);
#25395=ADVANCED_FACE('',(#3442),#24140,.F.);
#25396=ADVANCED_FACE('',(#3443),#2111,.F.);
#25397=ADVANCED_FACE('',(#3444),#2112,.T.);
#25398=ADVANCED_FACE('',(#3445),#2113,.T.);
#25399=ADVANCED_FACE('',(#3446),#2114,.F.);
#25400=ADVANCED_FACE('',(#3447),#2115,.F.);
#25401=ADVANCED_FACE('',(#3448),#2116,.F.);
#25402=ADVANCED_FACE('',(#3449),#2117,.F.);
#25403=ADVANCED_FACE('',(#3450),#24141,.T.);
#25404=ADVANCED_FACE('',(#3451),#2118,.T.);
#25405=ADVANCED_FACE('',(#3452,#1426),#24142,.T.);
#25685=CLOSED_SHELL('',(#25306,#25307,#25308,#25309,#25310,#25311,#25312,
#25313,#25314,#25315,#25316,#25317,#25318,#25319,#25320,#25321,#25322,#25323,
#25324,#25325,#25326));
#25686=CLOSED_SHELL('',(#25327,#25328,#25329,#25330,#25331,#25332,#25333,
#25334,#25335,#25336,#25337,#25338,#25339,#25340,#25341,#25342,#25343,#25344,
#25345,#25346,#25347,#25348,#25349,#25350,#25351,#25352,#25353,#25354,#25355,
#25356,#25357,#25358,#25359,#25360,#25361,#25362,#25363,#25364,#25365,#25366,
#25367,#25368,#25369,#25370,#25371,#25372,#25373,#25374,#25375,#25376,#25377,
#25378,#25379,#25380,#25381,#25382,#25383,#25384,#25385,#25386,#25387,#25388,
#25389,#25390,#25391,#25392,#25393,#25394,#25395,#25396,#25397,#25398,#25399,
#25400,#25401,#25402,#25403,#25404,#25405));
#28001=AXIS2_PLACEMENT_3D('',#64183,#34155,#34156);
#28002=AXIS2_PLACEMENT_3D('',#64184,#34157,#34158);
#28003=AXIS2_PLACEMENT_3D('',#64189,#34160,#34161);
#28004=AXIS2_PLACEMENT_3D('',#64192,#34163,#34164);
#28005=AXIS2_PLACEMENT_3D('',#64193,#34165,#34166);
#28006=AXIS2_PLACEMENT_3D('',#64196,#34167,#34168);
#28007=AXIS2_PLACEMENT_3D('',#64199,#34171,#34172);
#28008=AXIS2_PLACEMENT_3D('',#64202,#34173,#34174);
#28009=AXIS2_PLACEMENT_3D('',#64204,#34175,#34176);
#28010=AXIS2_PLACEMENT_3D('',#64206,#34177,#34178);
#28011=AXIS2_PLACEMENT_3D('',#64207,#34179,#34180);
#28012=AXIS2_PLACEMENT_3D('',#64208,#34181,#34182);
#28013=AXIS2_PLACEMENT_3D('',#64211,#34183,#34184);
#28014=AXIS2_PLACEMENT_3D('',#64213,#34185,#34186);
#28015=AXIS2_PLACEMENT_3D('',#64215,#34187,#34188);
#28016=AXIS2_PLACEMENT_3D('',#64216,#34189,#34190);
#28017=AXIS2_PLACEMENT_3D('',#64217,#34191,#34192);
#28018=AXIS2_PLACEMENT_3D('',#64220,#34193,#34194);
#28019=AXIS2_PLACEMENT_3D('',#64223,#34197,#34198);
#28020=AXIS2_PLACEMENT_3D('',#64228,#34201,#34202);
#28021=AXIS2_PLACEMENT_3D('',#64229,#34203,#34204);
#28022=AXIS2_PLACEMENT_3D('',#64232,#34206,#34207);
#28023=AXIS2_PLACEMENT_3D('',#64233,#34208,#34209);
#28024=AXIS2_PLACEMENT_3D('',#64236,#34211,#34212);
#28025=AXIS2_PLACEMENT_3D('',#64237,#34213,#34214);
#28026=AXIS2_PLACEMENT_3D('',#64239,#34215,#34216);
#28027=AXIS2_PLACEMENT_3D('',#64241,#34218,#34219);
#28028=AXIS2_PLACEMENT_3D('',#64243,#34220,#34221);
#28029=AXIS2_PLACEMENT_3D('',#64245,#34223,#34224);
#28030=AXIS2_PLACEMENT_3D('',#64246,#34225,#34226);
#28031=AXIS2_PLACEMENT_3D('',#64248,#34227,#34228);
#28032=AXIS2_PLACEMENT_3D('',#64252,#34231,#34232);
#28033=AXIS2_PLACEMENT_3D('',#64331,#34234,#34235);
#28034=AXIS2_PLACEMENT_3D('',#64335,#34237,#34238);
#28035=AXIS2_PLACEMENT_3D('',#64337,#34240,#34241);
#28036=AXIS2_PLACEMENT_3D('',#64340,#34244,#34245);
#28037=AXIS2_PLACEMENT_3D('',#64343,#34247,#34248);
#28038=AXIS2_PLACEMENT_3D('',#64344,#34249,#34250);
#28039=AXIS2_PLACEMENT_3D('',#64345,#34251,#34252);
#28040=AXIS2_PLACEMENT_3D('',#64347,#34253,#34254);
#28041=AXIS2_PLACEMENT_3D('',#64348,#34255,#34256);
#28042=AXIS2_PLACEMENT_3D('',#64350,#34257,#34258);
#28043=AXIS2_PLACEMENT_3D('',#64352,#34260,#34261);
#28044=AXIS2_PLACEMENT_3D('',#64354,#34262,#34263);
#28045=AXIS2_PLACEMENT_3D('',#64355,#34264,#34265);
#28046=AXIS2_PLACEMENT_3D('',#64357,#34266,#34267);
#28047=AXIS2_PLACEMENT_3D('',#64359,#34269,#34270);
#28048=AXIS2_PLACEMENT_3D('',#64360,#34271,#34272);
#28049=AXIS2_PLACEMENT_3D('',#64361,#34273,#34274);
#28050=AXIS2_PLACEMENT_3D('',#64362,#34275,#34276);
#28051=AXIS2_PLACEMENT_3D('',#64365,#34277,#34278);
#28052=AXIS2_PLACEMENT_3D('',#64396,#34279,#34280);
#28053=AXIS2_PLACEMENT_3D('',#64408,#34286,#34287);
#28054=AXIS2_PLACEMENT_3D('',#64409,#34288,#34289);
#28055=AXIS2_PLACEMENT_3D('',#64453,#34291,#34292);
#28056=AXIS2_PLACEMENT_3D('',#64455,#34293,#34294);
#28057=AXIS2_PLACEMENT_3D('',#64458,#34296,#34297);
#28058=AXIS2_PLACEMENT_3D('',#64459,#34298,#34299);
#28059=AXIS2_PLACEMENT_3D('',#64461,#34300,#34301);
#28060=AXIS2_PLACEMENT_3D('',#64462,#34302,#34303);
#28061=AXIS2_PLACEMENT_3D('',#64465,#34305,#34306);
#28062=AXIS2_PLACEMENT_3D('',#64466,#34307,#34308);
#28063=AXIS2_PLACEMENT_3D('',#64468,#34310,#34311);
#28064=AXIS2_PLACEMENT_3D('',#64479,#34317,#34318);
#28065=AXIS2_PLACEMENT_3D('',#64481,#34319,#34320);
#28066=AXIS2_PLACEMENT_3D('',#64488,#34324,#34325);
#28067=AXIS2_PLACEMENT_3D('',#64489,#34326,#34327);
#28068=AXIS2_PLACEMENT_3D('',#64490,#34328,#34329);
#28069=AXIS2_PLACEMENT_3D('',#64491,#34330,#34331);
#28070=AXIS2_PLACEMENT_3D('',#64492,#34332,#34333);
#28071=AXIS2_PLACEMENT_3D('',#64494,#34334,#34335);
#28072=AXIS2_PLACEMENT_3D('',#64496,#34336,#34337);
#28073=AXIS2_PLACEMENT_3D('',#64498,#34338,#34339);
#28074=AXIS2_PLACEMENT_3D('',#64500,#34340,#34341);
#28075=AXIS2_PLACEMENT_3D('',#64502,#34342,#34343);
#28076=AXIS2_PLACEMENT_3D('',#64504,#34344,#34345);
#28077=AXIS2_PLACEMENT_3D('',#64506,#34346,#34347);
#28078=AXIS2_PLACEMENT_3D('',#64508,#34348,#34349);
#28079=AXIS2_PLACEMENT_3D('',#64509,#34350,#34351);
#28080=AXIS2_PLACEMENT_3D('',#64511,#34352,#34353);
#28081=AXIS2_PLACEMENT_3D('',#64518,#34357,#34358);
#28082=AXIS2_PLACEMENT_3D('',#64519,#34359,#34360);
#28083=AXIS2_PLACEMENT_3D('',#64530,#34363,#34364);
#28084=AXIS2_PLACEMENT_3D('',#64542,#34367,#34368);
#28085=AXIS2_PLACEMENT_3D('',#64567,#34371,#34372);
#28086=AXIS2_PLACEMENT_3D('',#64568,#34373,#34374);
#28087=AXIS2_PLACEMENT_3D('',#64571,#34375,#34376);
#28088=AXIS2_PLACEMENT_3D('',#64666,#34378,#34379);
#28089=AXIS2_PLACEMENT_3D('',#64671,#34382,#34383);
#28090=AXIS2_PLACEMENT_3D('',#64674,#34386,#34387);
#28091=AXIS2_PLACEMENT_3D('',#64676,#34389,#34390);
#28092=AXIS2_PLACEMENT_3D('',#64678,#34392,#34393);
#28093=AXIS2_PLACEMENT_3D('',#64680,#34395,#34396);
#28094=AXIS2_PLACEMENT_3D('',#64682,#34398,#34399);
#28095=AXIS2_PLACEMENT_3D('',#64683,#34400,#34401);
#28096=AXIS2_PLACEMENT_3D('',#64684,#34402,#34403);
#28097=AXIS2_PLACEMENT_3D('',#64687,#34404,#34405);
#28098=AXIS2_PLACEMENT_3D('',#64690,#34408,#34409);
#28099=AXIS2_PLACEMENT_3D('',#64693,#34410,#34411);
#28100=AXIS2_PLACEMENT_3D('',#64696,#34414,#34415);
#28101=AXIS2_PLACEMENT_3D('',#64700,#34417,#34418);
#28102=AXIS2_PLACEMENT_3D('',#64702,#34420,#34421);
#28103=AXIS2_PLACEMENT_3D('',#64704,#34422,#34423);
#28104=AXIS2_PLACEMENT_3D('',#64706,#34425,#34426);
#28105=AXIS2_PLACEMENT_3D('',#64707,#34427,#34428);
#28106=AXIS2_PLACEMENT_3D('',#64708,#34429,#34430);
#28107=AXIS2_PLACEMENT_3D('',#64711,#34432,#34433);
#28108=AXIS2_PLACEMENT_3D('',#64712,#34434,#34435);
#28109=AXIS2_PLACEMENT_3D('',#64713,#34436,#34437);
#28110=AXIS2_PLACEMENT_3D('',#64714,#34438,#34439);
#28111=AXIS2_PLACEMENT_3D('',#64715,#34440,#34441);
#28112=AXIS2_PLACEMENT_3D('',#64716,#34442,#34443);
#28113=AXIS2_PLACEMENT_3D('',#64736,#34444,#34445);
#28114=AXIS2_PLACEMENT_3D('',#64740,#34447,#34448);
#28115=AXIS2_PLACEMENT_3D('',#64744,#34450,#34451);
#28116=AXIS2_PLACEMENT_3D('',#64748,#34453,#34454);
#28117=AXIS2_PLACEMENT_3D('',#64752,#34456,#34457);
#28118=AXIS2_PLACEMENT_3D('',#64756,#34459,#34460);
#28119=AXIS2_PLACEMENT_3D('',#64760,#34462,#34463);
#28120=AXIS2_PLACEMENT_3D('',#64764,#34465,#34466);
#28121=AXIS2_PLACEMENT_3D('',#64770,#34469,#34470);
#28122=AXIS2_PLACEMENT_3D('',#64772,#34471,#34472);
#28123=AXIS2_PLACEMENT_3D('',#64776,#34474,#34475);
#28124=AXIS2_PLACEMENT_3D('',#64777,#34476,#34477);
#28125=AXIS2_PLACEMENT_3D('',#64780,#34478,#34479);
#28126=AXIS2_PLACEMENT_3D('',#64784,#34481,#34482);
#28127=AXIS2_PLACEMENT_3D('',#64786,#34483,#34484);
#28128=AXIS2_PLACEMENT_3D('',#64790,#34486,#34487);
#28129=AXIS2_PLACEMENT_3D('',#64794,#34489,#34490);
#28130=AXIS2_PLACEMENT_3D('',#64796,#34491,#34492);
#28131=AXIS2_PLACEMENT_3D('',#64799,#34494,#34495);
#28132=AXIS2_PLACEMENT_3D('',#64802,#34496,#34497);
#28133=AXIS2_PLACEMENT_3D('',#64806,#34499,#34500);
#28134=AXIS2_PLACEMENT_3D('',#64808,#34501,#34502);
#28135=AXIS2_PLACEMENT_3D('',#64811,#34504,#34505);
#28136=AXIS2_PLACEMENT_3D('',#64812,#34506,#34507);
#28137=AXIS2_PLACEMENT_3D('',#64815,#34508,#34509);
#28138=AXIS2_PLACEMENT_3D('',#64819,#34511,#34512);
#28139=AXIS2_PLACEMENT_3D('',#64823,#34514,#34515);
#28140=AXIS2_PLACEMENT_3D('',#64827,#34517,#34518);
#28141=AXIS2_PLACEMENT_3D('',#64829,#34520,#34521);
#28142=AXIS2_PLACEMENT_3D('',#64832,#34524,#34525);
#28143=AXIS2_PLACEMENT_3D('',#64834,#34527,#34528);
#28144=AXIS2_PLACEMENT_3D('',#64836,#34530,#34531);
#28145=AXIS2_PLACEMENT_3D('',#64838,#34533,#34534);
#28146=AXIS2_PLACEMENT_3D('',#64840,#34536,#34537);
#28147=AXIS2_PLACEMENT_3D('',#64842,#34539,#34540);
#28148=AXIS2_PLACEMENT_3D('',#64844,#34542,#34543);
#28149=AXIS2_PLACEMENT_3D('',#64845,#34544,#34545);
#28150=AXIS2_PLACEMENT_3D('',#64849,#34547,#34548);
#28151=AXIS2_PLACEMENT_3D('',#64851,#34550,#34551);
#28152=AXIS2_PLACEMENT_3D('',#64855,#34554,#34555);
#28153=AXIS2_PLACEMENT_3D('',#64858,#34557,#34558);
#28154=AXIS2_PLACEMENT_3D('',#64859,#34559,#34560);
#28155=AXIS2_PLACEMENT_3D('',#64865,#34564,#34565);
#28156=AXIS2_PLACEMENT_3D('',#64868,#34567,#34568);
#28157=AXIS2_PLACEMENT_3D('',#64869,#34569,#34570);
#28158=AXIS2_PLACEMENT_3D('',#64872,#34572,#34573);
#28159=AXIS2_PLACEMENT_3D('',#64873,#34574,#34575);
#28160=AXIS2_PLACEMENT_3D('',#64877,#34578,#34579);
#28161=AXIS2_PLACEMENT_3D('',#64880,#34581,#34582);
#28162=AXIS2_PLACEMENT_3D('',#64881,#34583,#34584);
#28163=AXIS2_PLACEMENT_3D('',#64885,#34587,#34588);
#28164=AXIS2_PLACEMENT_3D('',#64886,#34589,#34590);
#28165=AXIS2_PLACEMENT_3D('',#64887,#34591,#34592);
#28166=AXIS2_PLACEMENT_3D('',#64888,#34593,#34594);
#28167=AXIS2_PLACEMENT_3D('',#64889,#34595,#34596);
#28168=AXIS2_PLACEMENT_3D('',#64890,#34597,#34598);
#28169=AXIS2_PLACEMENT_3D('',#64893,#34599,#34600);
#28170=AXIS2_PLACEMENT_3D('',#64897,#34602,#34603);
#28171=AXIS2_PLACEMENT_3D('',#64899,#34604,#34605);
#28172=AXIS2_PLACEMENT_3D('',#64902,#34607,#34608);
#28173=AXIS2_PLACEMENT_3D('',#64903,#34609,#34610);
#28174=AXIS2_PLACEMENT_3D('',#64906,#34613,#34614);
#28175=AXIS2_PLACEMENT_3D('',#64908,#34616,#34617);
#28176=AXIS2_PLACEMENT_3D('',#64910,#34619,#34620);
#28177=AXIS2_PLACEMENT_3D('',#64912,#34622,#34623);
#28178=AXIS2_PLACEMENT_3D('',#64914,#34625,#34626);
#28179=AXIS2_PLACEMENT_3D('',#64915,#34627,#34628);
#28180=AXIS2_PLACEMENT_3D('',#64921,#34632,#34633);
#28181=AXIS2_PLACEMENT_3D('',#64924,#34635,#34636);
#28182=AXIS2_PLACEMENT_3D('',#64925,#34637,#34638);
#28183=AXIS2_PLACEMENT_3D('',#64928,#34640,#34641);
#28184=AXIS2_PLACEMENT_3D('',#64929,#34642,#34643);
#28185=AXIS2_PLACEMENT_3D('',#64933,#34646,#34647);
#28186=AXIS2_PLACEMENT_3D('',#64935,#34648,#34649);
#28187=AXIS2_PLACEMENT_3D('',#64937,#34651,#34652);
#28188=AXIS2_PLACEMENT_3D('',#64938,#34653,#34654);
#28189=AXIS2_PLACEMENT_3D('',#64939,#34655,#34656);
#28190=AXIS2_PLACEMENT_3D('',#64940,#34657,#34658);
#28191=AXIS2_PLACEMENT_3D('',#64944,#34660,#34661);
#28192=AXIS2_PLACEMENT_3D('',#64946,#34663,#34664);
#28193=AXIS2_PLACEMENT_3D('',#64950,#34667,#34668);
#28194=AXIS2_PLACEMENT_3D('',#64953,#34670,#34671);
#28195=AXIS2_PLACEMENT_3D('',#64954,#34672,#34673);
#28196=AXIS2_PLACEMENT_3D('',#64973,#34675,#34676);
#28197=AXIS2_PLACEMENT_3D('',#64977,#34679,#34680);
#28198=AXIS2_PLACEMENT_3D('',#64981,#34682,#34683);
#28199=AXIS2_PLACEMENT_3D('',#64983,#34685,#34686);
#28200=AXIS2_PLACEMENT_3D('',#64987,#34689,#34690);
#28201=AXIS2_PLACEMENT_3D('',#64990,#34692,#34693);
#28202=AXIS2_PLACEMENT_3D('',#64991,#34694,#34695);
#28203=AXIS2_PLACEMENT_3D('',#64995,#34698,#34699);
#28204=AXIS2_PLACEMENT_3D('',#64998,#34701,#34702);
#28205=AXIS2_PLACEMENT_3D('',#64999,#34703,#34704);
#28206=AXIS2_PLACEMENT_3D('',#65001,#34706,#34707);
#28207=AXIS2_PLACEMENT_3D('',#65022,#34709,#34710);
#28208=AXIS2_PLACEMENT_3D('',#65024,#34712,#34713);
#34155=DIRECTION('axis',(0.,0.,1.));
#34156=DIRECTION('refdir',(1.,0.,0.));
#34157=DIRECTION('center_axis',(1.,0.,0.));
#34158=DIRECTION('ref_axis',(0.,1.,0.));
#34159=DIRECTION('',(0.,0.,-1.));
#34160=DIRECTION('center_axis',(1.,0.,0.));
#34161=DIRECTION('ref_axis',(0.,-0.707106781186548,0.707106781186548));
#34162=DIRECTION('',(0.,0.,-1.));
#34163=DIRECTION('center_axis',(-1.,0.,0.));
#34164=DIRECTION('ref_axis',(0.,-0.707106781186548,0.707106781186548));
#34165=DIRECTION('center_axis',(-1.,0.,0.));
#34166=DIRECTION('ref_axis',(0.,1.,8.30073289439369E-17));
#34167=DIRECTION('center_axis',(1.,0.,0.));
#34168=DIRECTION('ref_axis',(0.,-0.707106781186548,0.707106781186548));
#34169=DIRECTION('',(0.707104308763575,0.,-0.707109253600875));
#34170=DIRECTION('',(-0.707104308763575,0.,-0.707109253600875));
#34171=DIRECTION('center_axis',(-1.,0.,0.));
#34172=DIRECTION('ref_axis',(0.,0.,1.));
#34173=DIRECTION('center_axis',(1.,0.,0.));
#34174=DIRECTION('ref_axis',(0.,1.,0.));
#34175=DIRECTION('center_axis',(1.,0.,0.));
#34176=DIRECTION('ref_axis',(0.,-0.707106781186548,0.707106781186548));
#34177=DIRECTION('center_axis',(1.,0.,0.));
#34178=DIRECTION('ref_axis',(0.,0.,-1.));
#34179=DIRECTION('center_axis',(1.,0.,0.));
#34180=DIRECTION('ref_axis',(0.,0.707106781186547,-0.707106781186547));
#34181=DIRECTION('center_axis',(-1.,0.,0.));
#34182=DIRECTION('ref_axis',(0.,0.,1.));
#34183=DIRECTION('center_axis',(1.,0.,0.));
#34184=DIRECTION('ref_axis',(0.,0.,-1.));
#34185=DIRECTION('center_axis',(1.,0.,0.));
#34186=DIRECTION('ref_axis',(0.,-0.707106781186548,0.707106781186548));
#34187=DIRECTION('center_axis',(1.,0.,0.));
#34188=DIRECTION('ref_axis',(0.,-1.,0.));
#34189=DIRECTION('center_axis',(1.,0.,0.));
#34190=DIRECTION('ref_axis',(0.,0.707106781186547,-0.707106781186547));
#34191=DIRECTION('center_axis',(-1.,0.,0.));
#34192=DIRECTION('ref_axis',(0.,0.707106781186547,-0.707106781186547));
#34193=DIRECTION('center_axis',(1.,0.,0.));
#34194=DIRECTION('ref_axis',(0.,0.707106781186547,-0.707106781186547));
#34195=DIRECTION('',(-1.,0.,0.));
#34196=DIRECTION('',(1.,0.,0.));
#34197=DIRECTION('center_axis',(-1.,0.,0.));
#34198=DIRECTION('ref_axis',(0.,0.707106781186547,-0.707106781186547));
#34199=DIRECTION('',(-1.,0.,0.));
#34200=DIRECTION('',(1.,0.,0.));
#34201=DIRECTION('center_axis',(1.,0.,0.));
#34202=DIRECTION('ref_axis',(0.,0.707106781186547,-0.707106781186547));
#34203=DIRECTION('center_axis',(-1.,0.,0.));
#34204=DIRECTION('ref_axis',(0.,0.963284345089114,0.2684832778894));
#34205=DIRECTION('',(-1.,0.,0.));
#34206=DIRECTION('center_axis',(1.,0.,0.));
#34207=DIRECTION('ref_axis',(0.,-1.,0.));
#34208=DIRECTION('center_axis',(-1.,0.,0.));
#34209=DIRECTION('ref_axis',(0.,-0.2684832778894,0.963284345089114));
#34210=DIRECTION('',(-1.,0.,0.));
#34211=DIRECTION('center_axis',(1.,0.,0.));
#34212=DIRECTION('ref_axis',(0.,0.,-1.));
#34213=DIRECTION('center_axis',(-1.,0.,0.));
#34214=DIRECTION('ref_axis',(0.,0.,-1.));
#34215=DIRECTION('center_axis',(1.,0.,0.));
#34216=DIRECTION('ref_axis',(0.,0.,-1.));
#34217=DIRECTION('',(1.,0.,0.));
#34218=DIRECTION('center_axis',(-1.,0.,0.));
#34219=DIRECTION('ref_axis',(0.,1.,0.));
#34220=DIRECTION('center_axis',(1.,0.,0.));
#34221=DIRECTION('ref_axis',(0.,1.,0.));
#34222=DIRECTION('',(1.,0.,0.));
#34223=DIRECTION('center_axis',(1.,0.,0.));
#34224=DIRECTION('ref_axis',(0.,1.,-1.61486985400023E-16));
#34225=DIRECTION('center_axis',(1.,0.,0.));
#34226=DIRECTION('ref_axis',(0.,-0.707106781186548,0.707106781186548));
#34227=DIRECTION('center_axis',(1.,0.,0.));
#34228=DIRECTION('ref_axis',(0.,-0.707106781186548,0.707106781186548));
#34229=DIRECTION('',(1.,0.,0.));
#34230=DIRECTION('',(-1.,0.,0.));
#34231=DIRECTION('center_axis',(1.,0.,0.));
#34232=DIRECTION('ref_axis',(0.,-0.707106781186548,0.707106781186548));
#34233=DIRECTION('',(-1.,0.,0.));
#34234=DIRECTION('center_axis',(1.,0.,0.));
#34235=DIRECTION('ref_axis',(0.,1.,-1.85037170770859E-16));
#34236=DIRECTION('',(-1.,0.,0.));
#34237=DIRECTION('center_axis',(1.,0.,0.));
#34238=DIRECTION('ref_axis',(0.,-0.707106781186548,0.707106781186548));
#34239=DIRECTION('',(1.,0.,0.));
#34240=DIRECTION('center_axis',(1.,0.,0.));
#34241=DIRECTION('ref_axis',(0.,1.,0.));
#34242=DIRECTION('',(0.,0.,1.));
#34243=DIRECTION('',(0.,0.,1.));
#34244=DIRECTION('center_axis',(0.,-1.,0.));
#34245=DIRECTION('ref_axis',(1.,0.,0.));
#34246=DIRECTION('',(0.,-1.,0.));
#34247=DIRECTION('center_axis',(0.,-1.,0.));
#34248=DIRECTION('ref_axis',(1.,0.,0.));
#34249=DIRECTION('center_axis',(0.,-1.,0.));
#34250=DIRECTION('ref_axis',(0.,0.,-1.));
#34251=DIRECTION('center_axis',(0.,1.,0.));
#34252=DIRECTION('ref_axis',(1.,0.,0.));
#34253=DIRECTION('center_axis',(0.,1.,0.));
#34254=DIRECTION('ref_axis',(1.,0.,0.));
#34255=DIRECTION('center_axis',(0.,1.,0.));
#34256=DIRECTION('ref_axis',(1.,0.,0.));
#34257=DIRECTION('center_axis',(0.,1.,0.));
#34258=DIRECTION('ref_axis',(1.,0.,0.));
#34259=DIRECTION('',(0.,1.,0.));
#34260=DIRECTION('center_axis',(0.,-1.,0.));
#34261=DIRECTION('ref_axis',(0.,0.,-1.));
#34262=DIRECTION('center_axis',(0.,1.,0.));
#34263=DIRECTION('ref_axis',(1.,0.,0.));
#34264=DIRECTION('center_axis',(0.,1.,0.));
#34265=DIRECTION('ref_axis',(1.,0.,0.));
#34266=DIRECTION('center_axis',(0.,-1.,0.));
#34267=DIRECTION('ref_axis',(1.,0.,0.));
#34268=DIRECTION('',(0.,1.,0.));
#34269=DIRECTION('center_axis',(0.,-1.,0.));
#34270=DIRECTION('ref_axis',(0.,0.,-1.));
#34271=DIRECTION('center_axis',(0.,-1.,0.));
#34272=DIRECTION('ref_axis',(0.,0.,-1.));
#34273=DIRECTION('center_axis',(0.,1.,0.));
#34274=DIRECTION('ref_axis',(5.0532154980743E-16,0.,-1.));
#34275=DIRECTION('center_axis',(0.,-1.,0.));
#34276=DIRECTION('ref_axis',(5.0532154980743E-16,0.,1.));
#34277=DIRECTION('center_axis',(0.,-1.,0.));
#34278=DIRECTION('ref_axis',(1.,0.,0.));
#34279=DIRECTION('center_axis',(0.,1.,0.));
#34280=DIRECTION('ref_axis',(1.,0.,0.));
#34281=DIRECTION('',(-0.707104308763575,0.,0.707109253600875));
#34282=DIRECTION('',(0.,0.,1.));
#34283=DIRECTION('',(1.,0.,0.));
#34284=DIRECTION('',(0.,0.,-1.));
#34285=DIRECTION('',(-1.,0.,0.));
#34286=DIRECTION('center_axis',(0.,1.,0.));
#34287=DIRECTION('ref_axis',(1.,0.,0.));
#34288=DIRECTION('center_axis',(0.,1.,0.));
#34289=DIRECTION('ref_axis',(1.,0.,0.));
#34290=DIRECTION('',(0.,1.,0.));
#34291=DIRECTION('center_axis',(0.,-1.,0.));
#34292=DIRECTION('ref_axis',(1.,0.,0.));
#34293=DIRECTION('center_axis',(0.,1.,0.));
#34294=DIRECTION('ref_axis',(1.,0.,0.));
#34295=DIRECTION('',(0.,-1.,0.));
#34296=DIRECTION('center_axis',(0.,-1.,0.));
#34297=DIRECTION('ref_axis',(1.,0.,0.));
#34298=DIRECTION('center_axis',(0.,1.,0.));
#34299=DIRECTION('ref_axis',(1.,0.,0.));
#34300=DIRECTION('center_axis',(0.,-1.,0.));
#34301=DIRECTION('ref_axis',(1.,0.,0.));
#34302=DIRECTION('center_axis',(0.,-1.,0.));
#34303=DIRECTION('ref_axis',(1.,0.,0.));
#34304=DIRECTION('',(0.,-1.,0.));
#34305=DIRECTION('center_axis',(0.,-1.,0.));
#34306=DIRECTION('ref_axis',(1.,0.,0.));
#34307=DIRECTION('center_axis',(0.,1.,0.));
#34308=DIRECTION('ref_axis',(1.,0.,0.));
#34309=DIRECTION('',(-1.,0.,0.));
#34310=DIRECTION('center_axis',(0.,1.,0.));
#34311=DIRECTION('ref_axis',(1.,0.,0.));
#34312=DIRECTION('',(0.707104308763575,0.,0.707109253600875));
#34313=DIRECTION('',(1.,0.,0.));
#34314=DIRECTION('',(0.,0.,-1.));
#34315=DIRECTION('',(-1.,0.,0.));
#34316=DIRECTION('',(0.,0.,1.));
#34317=DIRECTION('center_axis',(1.,0.,0.));
#34318=DIRECTION('ref_axis',(0.,1.,0.));
#34319=DIRECTION('center_axis',(-1.,0.,0.));
#34320=DIRECTION('ref_axis',(0.,-0.707106781186548,0.707106781186548));
#34321=DIRECTION('',(0.,-1.,0.));
#34322=DIRECTION('',(0.,0.,1.));
#34323=DIRECTION('',(0.,1.,0.));
#34324=DIRECTION('center_axis',(-1.,0.,0.));
#34325=DIRECTION('ref_axis',(0.,-0.707106781186548,0.707106781186548));
#34326=DIRECTION('center_axis',(1.,0.,0.));
#34327=DIRECTION('ref_axis',(0.,-0.707106781186548,0.707106781186548));
#34328=DIRECTION('center_axis',(-1.,0.,0.));
#34329=DIRECTION('ref_axis',(0.,-0.707106781186548,0.707106781186548));
#34330=DIRECTION('center_axis',(1.,0.,0.));
#34331=DIRECTION('ref_axis',(0.,-0.707106781186548,0.707106781186548));
#34332=DIRECTION('center_axis',(1.,0.,0.));
#34333=DIRECTION('ref_axis',(0.,1.,0.));
#34334=DIRECTION('center_axis',(1.,0.,0.));
#34335=DIRECTION('ref_axis',(0.,-0.707106781186548,0.707106781186548));
#34336=DIRECTION('center_axis',(1.,0.,0.));
#34337=DIRECTION('ref_axis',(0.,-1.,0.));
#34338=DIRECTION('center_axis',(1.,0.,0.));
#34339=DIRECTION('ref_axis',(0.,0.707106781186547,-0.707106781186547));
#34340=DIRECTION('center_axis',(1.,0.,0.));
#34341=DIRECTION('ref_axis',(0.,0.,1.));
#34342=DIRECTION('center_axis',(1.,0.,0.));
#34343=DIRECTION('ref_axis',(0.,-0.707106781186548,0.707106781186548));
#34344=DIRECTION('center_axis',(1.,0.,0.));
#34345=DIRECTION('ref_axis',(0.,0.,1.));
#34346=DIRECTION('center_axis',(1.,0.,0.));
#34347=DIRECTION('ref_axis',(0.,0.707106781186547,-0.707106781186547));
#34348=DIRECTION('center_axis',(1.,0.,0.));
#34349=DIRECTION('ref_axis',(0.,1.,0.));
#34350=DIRECTION('center_axis',(1.,0.,0.));
#34351=DIRECTION('ref_axis',(0.,-0.707106781186548,0.707106781186548));
#34352=DIRECTION('center_axis',(1.,0.,0.));
#34353=DIRECTION('ref_axis',(0.,-0.707106781186548,0.707106781186548));
#34354=DIRECTION('',(0.,-1.,0.));
#34355=DIRECTION('',(0.,0.,-1.));
#34356=DIRECTION('',(0.,1.,0.));
#34357=DIRECTION('center_axis',(1.,0.,0.));
#34358=DIRECTION('ref_axis',(0.,-0.707106781186548,0.707106781186548));
#34359=DIRECTION('center_axis',(1.,0.,0.));
#34360=DIRECTION('ref_axis',(0.,-0.707106781186548,0.707106781186548));
#34361=DIRECTION('',(1.,0.,0.));
#34362=DIRECTION('',(1.,0.,0.));
#34363=DIRECTION('center_axis',(1.,0.,0.));
#34364=DIRECTION('ref_axis',(0.,-0.707106781186548,0.707106781186548));
#34365=DIRECTION('',(-1.,0.,0.));
#34366=DIRECTION('',(-1.,0.,0.));
#34367=DIRECTION('center_axis',(1.,0.,0.));
#34368=DIRECTION('ref_axis',(0.,-0.707106781186548,0.707106781186548));
#34369=DIRECTION('',(1.,0.,0.));
#34370=DIRECTION('',(-1.,0.,0.));
#34371=DIRECTION('center_axis',(1.,0.,0.));
#34372=DIRECTION('ref_axis',(0.,-0.707106781186548,0.707106781186548));
#34373=DIRECTION('center_axis',(0.,-1.,0.));
#34374=DIRECTION('ref_axis',(-1.,0.,0.));
#34375=DIRECTION('center_axis',(0.,1.,0.));
#34376=DIRECTION('ref_axis',(-1.,0.,0.));
#34377=DIRECTION('',(0.,-1.,0.));
#34378=DIRECTION('center_axis',(0.,1.,0.));
#34379=DIRECTION('ref_axis',(-1.,0.,0.));
#34380=DIRECTION('',(0.,1.,0.));
#34381=DIRECTION('',(0.,-1.,0.));
#34382=DIRECTION('center_axis',(0.,1.,0.));
#34383=DIRECTION('ref_axis',(-1.,0.,0.));
#34384=DIRECTION('',(0.,1.,0.));
#34385=DIRECTION('',(0.,-1.,0.));
#34386=DIRECTION('center_axis',(0.,0.,1.));
#34387=DIRECTION('ref_axis',(1.,0.,0.));
#34388=DIRECTION('',(1.,0.,0.));
#34389=DIRECTION('center_axis',(0.,0.,1.));
#34390=DIRECTION('ref_axis',(1.,0.,0.));
#34391=DIRECTION('',(1.,0.,0.));
#34392=DIRECTION('center_axis',(0.,-1.,0.));
#34393=DIRECTION('ref_axis',(0.,0.,-1.));
#34394=DIRECTION('',(-1.,0.,0.));
#34395=DIRECTION('center_axis',(0.,-1.,0.));
#34396=DIRECTION('ref_axis',(0.,0.,-1.));
#34397=DIRECTION('',(-1.,0.,0.));
#34398=DIRECTION('center_axis',(0.,0.,-1.));
#34399=DIRECTION('ref_axis',(0.,-1.,0.));
#34400=DIRECTION('center_axis',(0.,0.,-1.));
#34401=DIRECTION('ref_axis',(0.,-1.,0.));
#34402=DIRECTION('center_axis',(-1.,0.,0.));
#34403=DIRECTION('ref_axis',(0.,-0.963284345089114,-0.2684832778894));
#34404=DIRECTION('center_axis',(1.,0.,0.));
#34405=DIRECTION('ref_axis',(0.,1.,0.));
#34406=DIRECTION('',(-1.,0.,0.));
#34407=DIRECTION('',(1.,0.,0.));
#34408=DIRECTION('center_axis',(-1.,0.,0.));
#34409=DIRECTION('ref_axis',(0.,0.2684832778894,-0.963284345089114));
#34410=DIRECTION('center_axis',(1.,0.,0.));
#34411=DIRECTION('ref_axis',(0.,0.,1.));
#34412=DIRECTION('',(-1.,0.,0.));
#34413=DIRECTION('',(1.,0.,0.));
#34414=DIRECTION('center_axis',(-1.,0.,0.));
#34415=DIRECTION('ref_axis',(0.,-1.,0.));
#34416=DIRECTION('',(1.,0.,0.));
#34417=DIRECTION('center_axis',(1.,0.,0.));
#34418=DIRECTION('ref_axis',(0.,-1.,0.));
#34419=DIRECTION('',(-1.,0.,0.));
#34420=DIRECTION('center_axis',(-1.,0.,0.));
#34421=DIRECTION('ref_axis',(0.,-0.707106781186548,0.707106781186547));
#34422=DIRECTION('center_axis',(1.,0.,0.));
#34423=DIRECTION('ref_axis',(0.,0.707106781186547,-0.707106781186547));
#34424=DIRECTION('',(-1.,0.,0.));
#34425=DIRECTION('center_axis',(-1.,0.,0.));
#34426=DIRECTION('ref_axis',(0.,0.707106781186547,-0.707106781186547));
#34427=DIRECTION('center_axis',(1.,0.,0.));
#34428=DIRECTION('ref_axis',(0.,0.707106781186547,-0.707106781186547));
#34429=DIRECTION('center_axis',(-1.,0.,0.));
#34430=DIRECTION('ref_axis',(0.,0.,1.));
#34431=DIRECTION('',(1.,0.,0.));
#34432=DIRECTION('center_axis',(1.,0.,0.));
#34433=DIRECTION('ref_axis',(0.,0.,1.));
#34434=DIRECTION('center_axis',(-1.,0.,0.));
#34435=DIRECTION('ref_axis',(0.,0.,1.));
#34436=DIRECTION('center_axis',(1.,0.,0.));
#34437=DIRECTION('ref_axis',(0.,-0.707106781186548,0.707106781186548));
#34438=DIRECTION('center_axis',(-1.,0.,0.));
#34439=DIRECTION('ref_axis',(0.,0.,1.));
#34440=DIRECTION('center_axis',(1.,0.,0.));
#34441=DIRECTION('ref_axis',(0.,-0.707106781186548,0.707106781186548));
#34442=DIRECTION('center_axis',(1.,0.,0.));
#34443=DIRECTION('ref_axis',(0.,-0.707106781186548,0.707106781186548));
#34444=DIRECTION('center_axis',(0.946028810149189,0.229160959873926,0.229160958361957));
#34445=DIRECTION('ref_axis',(0.0238519321546227,-0.754422194584299,0.655955972341971));
#34446=DIRECTION('',(-1.,0.,0.));
#34447=DIRECTION('center_axis',(-0.946028810160763,-0.229160959093836,-0.229160959094266));
#34448=DIRECTION('ref_axis',(0.00756181520526069,-0.722522721083779,0.691305819784915));
#34449=DIRECTION('',(-1.,0.,0.));
#34450=DIRECTION('center_axis',(1.,0.,0.));
#34451=DIRECTION('ref_axis',(0.,-0.707106781186548,0.707106781186548));
#34452=DIRECTION('',(-1.,0.,0.));
#34453=DIRECTION('center_axis',(-1.,0.,0.));
#34454=DIRECTION('ref_axis',(0.,-0.707106781186548,0.707106781186548));
#34455=DIRECTION('',(1.,0.,0.));
#34456=DIRECTION('center_axis',(1.,0.,0.));
#34457=DIRECTION('ref_axis',(0.,-0.707106781186548,0.707106781186548));
#34458=DIRECTION('',(-1.,0.,0.));
#34459=DIRECTION('center_axis',(-1.,0.,0.));
#34460=DIRECTION('ref_axis',(0.,-0.707106781186548,0.707106781186548));
#34461=DIRECTION('',(-1.,0.,0.));
#34462=DIRECTION('center_axis',(-1.,0.,0.));
#34463=DIRECTION('ref_axis',(0.,-0.707106781186548,0.707106781186548));
#34464=DIRECTION('',(1.,0.,0.));
#34465=DIRECTION('center_axis',(1.,0.,0.));
#34466=DIRECTION('ref_axis',(0.,-0.707106781186548,0.707106781186548));
#34467=DIRECTION('',(-1.,0.,0.));
#34468=DIRECTION('',(1.,0.,0.));
#34469=DIRECTION('center_axis',(0.500000000011387,0.612372435691271,0.612372435691021));
#34470=DIRECTION('ref_axis',(0.866025403777864,-0.353553390477781,-0.353553390724871));
#34471=DIRECTION('center_axis',(-0.5000000000114,0.612372435691098,0.612372435691183));
#34472=DIRECTION('ref_axis',(0.866025403777857,0.35355339068672,0.353553390515949));
#34473=DIRECTION('',(1.,0.,0.));
#34474=DIRECTION('center_axis',(0.500000000001143,-0.612372435695232,-0.612372435695424));
#34475=DIRECTION('ref_axis',(0.866025403783779,0.35355339057273,0.353553390615434));
#34476=DIRECTION('center_axis',(-0.500000000001141,-0.612372435695253,-0.612372435695405));
#34477=DIRECTION('ref_axis',(0.86602540378378,-0.353553390639258,-0.353553390548903));
#34478=DIRECTION('center_axis',(-0.855183382509445,-0.366511515698828,-0.366511515698828));
#34479=DIRECTION('ref_axis',(0.518325556267202,-0.604705968930477,-0.604705968930477));
#34480=DIRECTION('',(-1.,0.,0.));
#34481=DIRECTION('center_axis',(-0.855183382508489,-0.366511515700201,-0.366511515699686));
#34482=DIRECTION('ref_axis',(0.00559375624135859,-0.713591574246071,0.7005396313244));
#34483=DIRECTION('center_axis',(1.,0.,0.));
#34484=DIRECTION('ref_axis',(0.,-0.707106781186548,0.707106781186548));
#34485=DIRECTION('',(-1.,0.,0.));
#34486=DIRECTION('center_axis',(-1.,0.,0.));
#34487=DIRECTION('ref_axis',(0.,-0.707106781186548,0.707106781186548));
#34488=DIRECTION('',(1.,0.,0.));
#34489=DIRECTION('center_axis',(1.,0.,0.));
#34490=DIRECTION('ref_axis',(0.,-0.707106781186548,0.707106781186548));
#34491=DIRECTION('center_axis',(-0.829037572548623,0.395409094042037,0.395409094042541));
#34492=DIRECTION('ref_axis',(0.0360858435025385,-0.667803081109337,0.74346274739195));
#34493=DIRECTION('',(1.,0.,0.));
#34494=DIRECTION('center_axis',(0.829037572553119,-0.395409094037575,-0.395409094037575));
#34495=DIRECTION('ref_axis',(-0.559192903473597,-0.586218089410745,-0.586218089410745));
#34496=DIRECTION('center_axis',(0.500000000011394,-0.612372435691112,-0.612372435691174));
#34497=DIRECTION('ref_axis',(0.86602540377786,0.353553390446867,0.353553390755794));
#34498=DIRECTION('',(-1.,0.,0.));
#34499=DIRECTION('center_axis',(-0.500000000001142,0.612372435695436,0.612372435695221));
#34500=DIRECTION('ref_axis',(0.866025403783779,0.353553390611745,0.353553390576418));
#34501=DIRECTION('center_axis',(0.500000000001144,0.612372435695425,0.61237243569523));
#34502=DIRECTION('ref_axis',(0.866025403783778,-0.353553390710462,-0.353553390477703));
#34503=DIRECTION('',(-1.,0.,0.));
#34504=DIRECTION('center_axis',(-0.500000000011398,-0.61237243569113,-0.612372435691153));
#34505=DIRECTION('ref_axis',(0.866025403777858,-0.353553390837826,-0.35355339036484));
#34506=DIRECTION('center_axis',(1.,0.,0.));
#34507=DIRECTION('ref_axis',(0.,-0.707106781186548,0.707106781186548));
#34508=DIRECTION('center_axis',(-1.,0.,0.));
#34509=DIRECTION('ref_axis',(0.,-0.707106781186548,0.707106781186548));
#34510=DIRECTION('',(1.,0.,0.));
#34511=DIRECTION('center_axis',(-1.,0.,0.));
#34512=DIRECTION('ref_axis',(0.,-0.707106781186548,0.707106781186548));
#34513=DIRECTION('',(-1.,0.,0.));
#34514=DIRECTION('center_axis',(1.,0.,0.));
#34515=DIRECTION('ref_axis',(0.,-0.707106781186548,0.707106781186548));
#34516=DIRECTION('',(1.,0.,0.));
#34517=DIRECTION('center_axis',(1.,0.,0.));
#34518=DIRECTION('ref_axis',(0.,-0.707106781186548,0.707106781186548));
#34519=DIRECTION('',(1.,0.,0.));
#34520=DIRECTION('center_axis',(-1.,0.,0.));
#34521=DIRECTION('ref_axis',(0.,0.,1.));
#34522=DIRECTION('',(0.,-0.707106781186547,0.707106781186547));
#34523=DIRECTION('',(0.,-0.707106781186547,0.707106781186547));
#34524=DIRECTION('center_axis',(0.,-0.707106781186548,-0.707106781186548));
#34525=DIRECTION('ref_axis',(0.,-0.707106781186548,0.707106781186548));
#34526=DIRECTION('',(0.,-0.707106781186547,0.707106781186547));
#34527=DIRECTION('center_axis',(0.,-0.707106781186548,-0.707106781186548));
#34528=DIRECTION('ref_axis',(0.,-0.707106781186548,0.707106781186548));
#34529=DIRECTION('',(0.,-0.707106781186547,0.707106781186547));
#34530=DIRECTION('center_axis',(-1.,0.,0.));
#34531=DIRECTION('ref_axis',(0.,0.,1.));
#34532=DIRECTION('',(0.,-0.707106781186547,0.707106781186547));
#34533=DIRECTION('center_axis',(0.,0.707106781186548,0.707106781186548));
#34534=DIRECTION('ref_axis',(1.,0.,0.));
#34535=DIRECTION('',(0.,-0.707106781186547,0.707106781186547));
#34536=DIRECTION('center_axis',(1.,0.,0.));
#34537=DIRECTION('ref_axis',(0.,1.,0.));
#34538=DIRECTION('',(0.,-0.707106781186547,0.707106781186547));
#34539=DIRECTION('center_axis',(0.,-0.707106781186548,-0.707106781186548));
#34540=DIRECTION('ref_axis',(0.,-0.707106781186548,0.707106781186548));
#34541=DIRECTION('',(0.,-0.707106781186547,0.707106781186547));
#34542=DIRECTION('center_axis',(1.,0.,0.));
#34543=DIRECTION('ref_axis',(0.,1.,0.));
#34544=DIRECTION('center_axis',(-0.855183382508501,-0.366511515699929,-0.366511515699929));
#34545=DIRECTION('ref_axis',(-0.393923250037275,2.21791245245237E-17,0.919143336525958));
#34546=DIRECTION('',(0.,-0.707106781186547,0.707106781186547));
#34547=DIRECTION('center_axis',(0.855183382508501,0.366511515699929,0.366511515699929));
#34548=DIRECTION('ref_axis',(0.518325556268759,-0.60470596892981,-0.60470596892981));
#34549=DIRECTION('',(0.,-0.707106781186547,0.707106781186547));
#34550=DIRECTION('center_axis',(0.,-0.707106781186548,-0.707106781186548));
#34551=DIRECTION('ref_axis',(0.,-0.707106781186548,0.707106781186548));
#34552=DIRECTION('',(0.,-0.707106781186547,0.707106781186547));
#34553=DIRECTION('',(1.,0.,0.));
#34554=DIRECTION('center_axis',(0.855183382509445,0.366511515698828,0.366511515698828));
#34555=DIRECTION('ref_axis',(1.39157273869269E-18,0.707106781186548,-0.707106781186548));
#34556=DIRECTION('',(0.,-0.707106781186548,0.707106781186548));
#34557=DIRECTION('center_axis',(0.855183382509445,0.366511515698828,0.366511515698828));
#34558=DIRECTION('ref_axis',(0.518325556267202,-0.604705968930478,-0.604705968930478));
#34559=DIRECTION('center_axis',(0.,0.707106781186548,0.707106781186548));
#34560=DIRECTION('ref_axis',(1.,0.,0.));
#34561=DIRECTION('',(0.,-0.707106781186547,0.707106781186547));
#34562=DIRECTION('',(-1.,0.,0.));
#34563=DIRECTION('',(0.,-0.707106781186547,0.707106781186547));
#34564=DIRECTION('center_axis',(-0.829037572548639,0.395409094042272,0.395409094042272));
#34565=DIRECTION('ref_axis',(0.430491988667656,7.53182077044634E-18,0.902594398217143));
#34566=DIRECTION('',(0.,-0.707106781186547,0.707106781186547));
#34567=DIRECTION('center_axis',(0.82903757254862,-0.395409094041967,-0.395409094042617));
#34568=DIRECTION('ref_axis',(0.0128476572574178,-0.693451556770021,0.7203886979376));
#34569=DIRECTION('center_axis',(1.,0.,0.));
#34570=DIRECTION('ref_axis',(0.,1.,0.));
#34571=DIRECTION('',(0.,-0.707106781186547,0.707106781186547));
#34572=DIRECTION('center_axis',(-1.,0.,0.));
#34573=DIRECTION('ref_axis',(0.,-0.707106781186548,0.707106781186548));
#34574=DIRECTION('center_axis',(0.,0.707106781186548,0.707106781186548));
#34575=DIRECTION('ref_axis',(1.,0.,0.));
#34576=DIRECTION('',(0.,-0.707106781186547,0.707106781186547));
#34577=DIRECTION('',(-1.,0.,0.));
#34578=DIRECTION('center_axis',(-1.,0.,0.));
#34579=DIRECTION('ref_axis',(0.,0.,1.));
#34580=DIRECTION('',(0.,-0.707106781186547,0.707106781186547));
#34581=DIRECTION('center_axis',(1.,0.,0.));
#34582=DIRECTION('ref_axis',(0.,-0.707106781186548,0.707106781186548));
#34583=DIRECTION('center_axis',(0.,-0.707106781186548,-0.707106781186548));
#34584=DIRECTION('ref_axis',(0.,-0.707106781186548,0.707106781186548));
#34585=DIRECTION('',(0.,-0.707106781186547,0.707106781186547));
#34586=DIRECTION('',(1.,0.,0.));
#34587=DIRECTION('center_axis',(1.,0.,0.));
#34588=DIRECTION('ref_axis',(0.,1.,0.));
#34589=DIRECTION('center_axis',(-1.,0.,0.));
#34590=DIRECTION('ref_axis',(0.,-0.707106781186548,0.707106781186548));
#34591=DIRECTION('center_axis',(0.829037572553119,-0.395409094037575,-0.395409094037575));
#34592=DIRECTION('ref_axis',(-9.11250315044804E-18,-0.707106781186548,0.707106781186548));
#34593=DIRECTION('center_axis',(-0.829037572553119,0.395409094037575,0.395409094037575));
#34594=DIRECTION('ref_axis',(-0.559192903473597,-0.586218089410745,-0.586218089410745));
#34595=DIRECTION('center_axis',(1.,0.,0.));
#34596=DIRECTION('ref_axis',(0.,-0.707106781186548,0.707106781186548));
#34597=DIRECTION('center_axis',(1.,0.,0.));
#34598=DIRECTION('ref_axis',(0.,-0.707106781186548,0.707106781186548));
#34599=DIRECTION('center_axis',(-0.500000000001105,0.612372435695761,0.612372435694926));
#34600=DIRECTION('ref_axis',(0.866025403783801,0.353553390633539,0.353553390554571));
#34601=DIRECTION('',(-1.,0.,0.));
#34602=DIRECTION('center_axis',(0.500000000011393,-0.612372435691199,-0.612372435691088));
#34603=DIRECTION('ref_axis',(0.866025403777861,0.353553390281616,0.353553390921043));
#34604=DIRECTION('center_axis',(-0.500000000011371,-0.612372435691481,-0.612372435690824));
#34605=DIRECTION('ref_axis',(0.866025403777874,-0.353553389921635,-0.353553391280993));
#34606=DIRECTION('',(-1.,0.,0.));
#34607=DIRECTION('center_axis',(0.500000000001104,0.612372435695737,0.612372435694951));
#34608=DIRECTION('ref_axis',(0.866025403783801,-0.353553390620861,-0.353553390567248));
#34609=DIRECTION('center_axis',(-0.500000000011394,0.612372435691143,0.612372435691143));
#34610=DIRECTION('ref_axis',(0.774596669232069,-4.54116170797946E-18,0.632455532045206));
#34611=DIRECTION('',(0.,-0.707106781186547,0.707106781186547));
#34612=DIRECTION('',(0.,-0.707106781186547,0.707106781186547));
#34613=DIRECTION('center_axis',(0.500000000011394,0.612372435691143,0.612372435691143));
#34614=DIRECTION('ref_axis',(0.774596669232069,4.54116170797946E-18,-0.632455532045206));
#34615=DIRECTION('',(0.,-0.707106781186547,0.707106781186547));
#34616=DIRECTION('center_axis',(0.,0.707106781186548,0.707106781186548));
#34617=DIRECTION('ref_axis',(1.,0.,0.));
#34618=DIRECTION('',(0.,-0.707106781186547,0.707106781186547));
#34619=DIRECTION('center_axis',(0.500000000001135,-0.612372435695331,-0.612372435695331));
#34620=DIRECTION('ref_axis',(-1.13185083784068E-17,-0.707106781186548,0.707106781186548));
#34621=DIRECTION('',(0.,-0.707106781186547,0.707106781186547));
#34622=DIRECTION('center_axis',(-0.500000000001135,-0.612372435695331,-0.612372435695331));
#34623=DIRECTION('ref_axis',(1.13185083784068E-17,-0.707106781186548,0.707106781186548));
#34624=DIRECTION('',(0.,-0.707106781186547,0.707106781186547));
#34625=DIRECTION('center_axis',(0.,0.707106781186548,0.707106781186548));
#34626=DIRECTION('ref_axis',(1.,0.,0.));
#34627=DIRECTION('center_axis',(0.,-0.707106781186548,-0.707106781186548));
#34628=DIRECTION('ref_axis',(0.,-0.707106781186548,0.707106781186548));
#34629=DIRECTION('',(0.,-0.707106781186547,0.707106781186547));
#34630=DIRECTION('',(1.,0.,0.));
#34631=DIRECTION('',(0.,-0.707106781186547,0.707106781186547));
#34632=DIRECTION('center_axis',(0.500000000001135,0.612372435695331,0.612372435695331));
#34633=DIRECTION('ref_axis',(0.774596669240545,3.67462033374012E-17,-0.632455532034825));
#34634=DIRECTION('',(0.,-0.707106781186547,0.707106781186547));
#34635=DIRECTION('center_axis',(-0.5000000000011,-0.612372435694895,-0.612372435695796));
#34636=DIRECTION('ref_axis',(0.866025403783803,-0.353553390588746,-0.353553390599358));
#34637=DIRECTION('center_axis',(-0.500000000001135,0.612372435695331,0.612372435695331));
#34638=DIRECTION('ref_axis',(0.774596669240545,-3.67462033374012E-17,0.632455532034825));
#34639=DIRECTION('',(0.,-0.707106781186547,0.707106781186547));
#34640=DIRECTION('center_axis',(0.500000000001106,-0.612372435694935,-0.612372435695752));
#34641=DIRECTION('ref_axis',(0.8660254037838,0.353553390608041,0.35355339058007));
#34642=DIRECTION('center_axis',(0.,-0.707106781186548,-0.707106781186548));
#34643=DIRECTION('ref_axis',(0.,-0.707106781186548,0.707106781186548));
#34644=DIRECTION('',(0.,-0.707106781186547,0.707106781186547));
#34645=DIRECTION('',(1.,0.,0.));
#34646=DIRECTION('center_axis',(-0.500000000011394,-0.612372435691143,-0.612372435691143));
#34647=DIRECTION('ref_axis',(6.99246513044329E-19,-0.707106781186548,0.707106781186548));
#34648=DIRECTION('center_axis',(0.500000000011403,0.612372435691209,0.61237243569107));
#34649=DIRECTION('ref_axis',(0.866025403777855,-0.353553390419331,-0.353553390783343));
#34650=DIRECTION('',(0.,-0.707106781186547,0.707106781186547));
#34651=DIRECTION('center_axis',(0.500000000011394,-0.612372435691143,-0.612372435691143));
#34652=DIRECTION('ref_axis',(-6.99246513044329E-19,-0.707106781186548,0.707106781186548));
#34653=DIRECTION('center_axis',(-0.500000000011383,0.612372435690964,0.612372435691331));
#34654=DIRECTION('ref_axis',(0.866025403777866,0.353553390491497,0.35355339071115));
#34655=DIRECTION('center_axis',(1.,0.,0.));
#34656=DIRECTION('ref_axis',(0.,-0.707106781186548,0.707106781186548));
#34657=DIRECTION('center_axis',(-0.946028810160758,-0.229160959094061,-0.229160959094061));
#34658=DIRECTION('ref_axis',(-0.235425987742297,-1.02571817929429E-18,0.971892280191362));
#34659=DIRECTION('',(0.,-0.707106781186547,0.707106781186547));
#34660=DIRECTION('center_axis',(0.946028810160763,0.229160959093891,0.229160959094211));
#34661=DIRECTION('ref_axis',(0.0242942123304843,-0.75526323419992,0.654971173650504));
#34662=DIRECTION('',(0.,-0.707106781186548,0.707106781186548));
#34663=DIRECTION('center_axis',(0.,-0.707106781186548,-0.707106781186548));
#34664=DIRECTION('ref_axis',(0.,-0.707106781186548,0.707106781186548));
#34665=DIRECTION('',(0.,-0.707106781186547,0.707106781186547));
#34666=DIRECTION('',(1.,0.,0.));
#34667=DIRECTION('center_axis',(0.946028810171404,0.229160959072088,0.229160959072088));
#34668=DIRECTION('ref_axis',(7.7304114234421E-18,0.707106781186548,-0.707106781186548));
#34669=DIRECTION('',(0.,-0.707106781186547,0.707106781186547));
#34670=DIRECTION('center_axis',(-0.946028810149188,-0.229160959860184,-0.229160958375702));
#34671=DIRECTION('ref_axis',(0.00521156151953889,-0.717772603447844,0.696258091059797));
#34672=DIRECTION('center_axis',(0.,-0.707106781186548,0.707106781186548));
#34673=DIRECTION('ref_axis',(0.587785252292473,-0.572061402817684,-0.572061402817684));
#34674=DIRECTION('',(0.,-0.707106781186547,0.707106781186547));
#34675=DIRECTION('center_axis',(0.,0.707106781186548,0.707106781186548));
#34676=DIRECTION('ref_axis',(1.,0.,0.));
#34677=DIRECTION('',(0.,-0.707106781186547,0.707106781186547));
#34678=DIRECTION('',(-1.,0.,0.));
#34679=DIRECTION('center_axis',(-1.,0.,0.));
#34680=DIRECTION('ref_axis',(0.,0.,1.));
#34681=DIRECTION('',(0.,-0.707106781186548,0.707106781186548));
#34682=DIRECTION('center_axis',(-1.,0.,0.));
#34683=DIRECTION('ref_axis',(0.,-0.707106781186548,0.707106781186548));
#34684=DIRECTION('',(0.,-0.707106781186547,0.707106781186547));
#34685=DIRECTION('center_axis',(0.,0.707106781186548,0.707106781186548));
#34686=DIRECTION('ref_axis',(1.,0.,0.));
#34687=DIRECTION('',(0.,-0.707106781186548,0.707106781186548));
#34688=DIRECTION('',(1.,0.,0.));
#34689=DIRECTION('center_axis',(-1.,0.,0.));
#34690=DIRECTION('ref_axis',(0.,0.,1.));
#34691=DIRECTION('',(0.,-0.707106781186547,0.707106781186547));
#34692=DIRECTION('center_axis',(1.,0.,0.));
#34693=DIRECTION('ref_axis',(0.,-0.707106781186548,0.707106781186548));
#34694=DIRECTION('center_axis',(0.,-0.707106781186548,-0.707106781186548));
#34695=DIRECTION('ref_axis',(0.,-0.707106781186548,0.707106781186548));
#34696=DIRECTION('',(0.,-0.707106781186547,0.707106781186547));
#34697=DIRECTION('',(1.,0.,0.));
#34698=DIRECTION('center_axis',(1.,0.,0.));
#34699=DIRECTION('ref_axis',(0.,1.,0.));
#34700=DIRECTION('',(0.,-0.707106781186548,0.707106781186548));
#34701=DIRECTION('center_axis',(-1.,0.,0.));
#34702=DIRECTION('ref_axis',(0.,-0.707106781186548,0.707106781186548));
#34703=DIRECTION('center_axis',(0.,-0.707106781186548,-0.707106781186548));
#34704=DIRECTION('ref_axis',(0.,-0.707106781186548,0.707106781186548));
#34705=DIRECTION('',(1.,0.,0.));
#34706=DIRECTION('center_axis',(0.,-0.707106781186548,0.707106781186548));
#34707=DIRECTION('ref_axis',(0.,-0.707106781186547,-0.707106781186547));
#34708=DIRECTION('',(0.,-0.707106781186547,0.707106781186547));
#34709=DIRECTION('center_axis',(0.,-0.707106781186548,-0.707106781186548));
#34710=DIRECTION('ref_axis',(0.,-0.707106781186548,0.707106781186548));
#34711=DIRECTION('',(-1.,0.,0.));
#34712=DIRECTION('center_axis',(1.,0.,0.));
#34713=DIRECTION('ref_axis',(0.,-0.707106781186548,0.707106781186548));
#64183=CARTESIAN_POINT('',(0.,0.,0.));
#64184=CARTESIAN_POINT('Origin',(39.,-9.19238815542512,9.19238815542512));
#64185=CARTESIAN_POINT('',(39.,0.1,-5.99916660878826));
#64186=CARTESIAN_POINT('',(39.,0.1,-25.9998076915965));
#64187=CARTESIAN_POINT('',(39.,0.1,4.59619407771256));
#64188=CARTESIAN_POINT('',(39.,0.1,25.9998076915965));
#64189=CARTESIAN_POINT('Origin',(39.,0.,0.));
#64190=CARTESIAN_POINT('',(39.,0.1,5.99916660878826));
#64191=CARTESIAN_POINT('',(39.,0.1,4.59619407771256));
#64192=CARTESIAN_POINT('Origin',(39.,0.,0.));
#64193=CARTESIAN_POINT('Origin',(38.25,0.,0.));
#64194=CARTESIAN_POINT('',(37.5,0.1,-27.4998181812171));
#64195=CARTESIAN_POINT('',(37.5,0.1,27.4998181812171));
#64196=CARTESIAN_POINT('Origin',(37.5,0.,0.));
#64197=CARTESIAN_POINT('',(38.25,0.1,26.7498129364068));
#64198=CARTESIAN_POINT('',(38.25,0.1,-26.7498129364068));
#64199=CARTESIAN_POINT('Origin',(-7.,-9.72271824131503,9.72271824131503));
#64200=CARTESIAN_POINT('',(-7.,10.0876161703348,14.3));
#64201=CARTESIAN_POINT('',(-7.,12.8747815515449,24.3));
#64202=CARTESIAN_POINT('Origin',(-7.,0.,22.5));
#64203=CARTESIAN_POINT('',(-7.,24.3,12.8747815515449));
#64204=CARTESIAN_POINT('Origin',(-7.,0.,0.));
#64205=CARTESIAN_POINT('',(-7.,14.3,10.0876161703348));
#64206=CARTESIAN_POINT('Origin',(-7.,22.5,0.));
#64207=CARTESIAN_POINT('Origin',(-7.,0.,0.));
#64208=CARTESIAN_POINT('Origin',(-7.,-9.72271824131503,9.72271824131503));
#64209=CARTESIAN_POINT('',(-7.,14.3,-10.0876161703348));
#64210=CARTESIAN_POINT('',(-7.,24.3,-12.8747815515449));
#64211=CARTESIAN_POINT('Origin',(-7.,22.5,0.));
#64212=CARTESIAN_POINT('',(-7.,12.8747815515449,-24.3));
#64213=CARTESIAN_POINT('Origin',(-7.,0.,0.));
#64214=CARTESIAN_POINT('',(-7.,10.0876161703348,-14.3));
#64215=CARTESIAN_POINT('Origin',(-7.,0.,-22.5));
#64216=CARTESIAN_POINT('Origin',(-7.,0.,0.));
#64217=CARTESIAN_POINT('Origin',(1.,0.,0.));
#64218=CARTESIAN_POINT('',(9.,10.0876161703348,-14.3));
#64219=CARTESIAN_POINT('',(9.,14.3,-10.0876161703348));
#64220=CARTESIAN_POINT('Origin',(9.,0.,0.));
#64221=CARTESIAN_POINT('',(1.,14.3,-10.0876161703348));
#64222=CARTESIAN_POINT('',(1.,10.0876161703348,-14.3));
#64223=CARTESIAN_POINT('Origin',(1.,0.,0.));
#64224=CARTESIAN_POINT('',(9.,10.0876161703348,14.3));
#64225=CARTESIAN_POINT('',(1.,10.0876161703348,14.3));
#64226=CARTESIAN_POINT('',(9.,14.3,10.0876161703348));
#64227=CARTESIAN_POINT('',(1.,14.3,10.0876161703348));
#64228=CARTESIAN_POINT('Origin',(9.,0.,0.));
#64229=CARTESIAN_POINT('Origin',(1.,0.,-22.5));
#64230=CARTESIAN_POINT('',(9.,12.8747815515449,-24.3));
#64231=CARTESIAN_POINT('',(1.,12.8747815515449,-24.3));
#64232=CARTESIAN_POINT('Origin',(9.,0.,-22.5));
#64233=CARTESIAN_POINT('Origin',(1.,22.5,0.));
#64234=CARTESIAN_POINT('',(9.,24.3,12.8747815515449));
#64235=CARTESIAN_POINT('',(1.,24.3,12.8747815515449));
#64236=CARTESIAN_POINT('Origin',(9.,22.5,0.));
#64237=CARTESIAN_POINT('Origin',(1.,22.5,0.));
#64238=CARTESIAN_POINT('',(9.,24.3,-12.8747815515449));
#64239=CARTESIAN_POINT('Origin',(9.,22.5,0.));
#64240=CARTESIAN_POINT('',(1.,24.3,-12.8747815515449));
#64241=CARTESIAN_POINT('Origin',(1.,0.,22.5));
#64242=CARTESIAN_POINT('',(9.,12.8747815515449,24.3));
#64243=CARTESIAN_POINT('Origin',(9.,0.,22.5));
#64244=CARTESIAN_POINT('',(1.,12.8747815515449,24.3));
#64245=CARTESIAN_POINT('Origin',(15.25,0.,0.));
#64246=CARTESIAN_POINT('Origin',(9.,0.,0.));
#64247=CARTESIAN_POINT('',(9.,0.1,27.4998181812171));
#64248=CARTESIAN_POINT('Origin',(9.,0.,0.));
#64249=CARTESIAN_POINT('',(15.25,0.1,27.4998181812171));
#64250=CARTESIAN_POINT('',(9.,0.1,-27.4998181812171));
#64251=CARTESIAN_POINT('',(15.25,0.1,-27.4998181812171));
#64252=CARTESIAN_POINT('Origin',(9.,0.,0.));
#64253=CARTESIAN_POINT('',(26.4377160017529,19.4454364826301,-19.4454364826301));
#64254=CARTESIAN_POINT('',(21.5,18.8745860881769,-20.));
#64255=CARTESIAN_POINT('Ctrl Pts',(26.4377160017535,19.4454364826275,-19.4454364826326));
#64256=CARTESIAN_POINT('Ctrl Pts',(26.4059901055805,19.5848952143129,-19.3059777509472));
#64257=CARTESIAN_POINT('Ctrl Pts',(26.3612673723032,19.7227284607851,-19.1650944052198));
#64258=CARTESIAN_POINT('Ctrl Pts',(26.1640017219762,20.169832853608,-18.6985071174812));
#64259=CARTESIAN_POINT('Ctrl Pts',(25.945163052824,20.4554595320486,-18.383121240662));
#64260=CARTESIAN_POINT('Ctrl Pts',(25.4583216143465,20.8332972173375,-17.9521176633326));
#64261=CARTESIAN_POINT('Ctrl Pts',(25.2031277311749,20.9737985255456,-17.7868382119765));
#64262=CARTESIAN_POINT('Ctrl Pts',(24.6276828245849,21.1637417254346,-17.5604063991252));
#64263=CARTESIAN_POINT('Ctrl Pts',(24.3071450917694,21.2132034355965,-17.5));
#64264=CARTESIAN_POINT('Ctrl Pts',(23.6928549082306,21.2132034355965,-17.5));
#64265=CARTESIAN_POINT('Ctrl Pts',(23.3723171754151,21.1637417254346,-17.5604063991252));
#64266=CARTESIAN_POINT('Ctrl Pts',(22.7968722688252,20.9737985255456,-17.7868382119765));
#64267=CARTESIAN_POINT('Ctrl Pts',(22.5416783856535,20.8332972173375,-17.9521176633326));
#64268=CARTESIAN_POINT('Ctrl Pts',(22.0548369471761,20.4554595320486,-18.383121240662));
#64269=CARTESIAN_POINT('Ctrl Pts',(21.8359982780239,20.169832853608,-18.6985071174812));
#64270=CARTESIAN_POINT('Ctrl Pts',(21.5586819382302,19.5412928441449,-19.3544362091167));
#64271=CARTESIAN_POINT('Ctrl Pts',(21.5,19.1981343317555,-19.6946580411449));
#64272=CARTESIAN_POINT('Ctrl Pts',(21.5,18.8745860881769,-20.));
#64273=CARTESIAN_POINT('Ctrl Pts',(21.5,18.8745860881769,-20.));
#64274=CARTESIAN_POINT('Ctrl Pts',(21.5,18.5112642482312,-20.3428774672885));
#64275=CARTESIAN_POINT('Ctrl Pts',(21.5732810359517,18.1082220917789,-20.7028459652353));
#64276=CARTESIAN_POINT('Ctrl Pts',(21.8751326101794,17.3199088998874,-21.3667099444405));
#64277=CARTESIAN_POINT('Ctrl Pts',(22.1019786827811,16.9344413423488,-21.6711549104462));
#64278=CARTESIAN_POINT('Ctrl Pts',(22.5800189982876,16.4058021284168,-22.0718427713117));
#64279=CARTESIAN_POINT('Ctrl Pts',(22.8176675360957,16.2001944002355,-22.222452745926));
#64280=CARTESIAN_POINT('Ctrl Pts',(23.2304377099712,15.976589433265,-22.3831860081774));
#64281=CARTESIAN_POINT('Ctrl Pts',(23.3774232617092,15.9159206638649,-22.4262333390977));
#64282=CARTESIAN_POINT('Ctrl Pts',(23.6826872283767,15.8333169759962,-22.4846329655715));
#64283=CARTESIAN_POINT('Ctrl Pts',(23.8409645128471,15.8113883008419,-22.5));
#64284=CARTESIAN_POINT('Ctrl Pts',(24.,15.8113883008419,-22.5));
#64285=CARTESIAN_POINT('Ctrl Pts',(24.1590354871529,15.8113883008419,-22.5));
#64286=CARTESIAN_POINT('Ctrl Pts',(24.3173127716233,15.8333169759962,-22.4846329655715));
#64287=CARTESIAN_POINT('Ctrl Pts',(24.6225767382908,15.9159206638649,-22.4262333390977));
#64288=CARTESIAN_POINT('Ctrl Pts',(24.7695622900288,15.976589433265,-22.3831860081774));
#64289=CARTESIAN_POINT('Ctrl Pts',(25.1823324639043,16.2001944002355,-22.222452745926));
#64290=CARTESIAN_POINT('Ctrl Pts',(25.4199810017124,16.4058021284168,-22.0718427713117));
#64291=CARTESIAN_POINT('Ctrl Pts',(25.8980213172189,16.9344413423488,-21.6711549104462));
#64292=CARTESIAN_POINT('Ctrl Pts',(26.1248673898206,17.3199088998874,-21.3667099444405));
#64293=CARTESIAN_POINT('Ctrl Pts',(26.4267189640483,18.1082220917789,-20.7028459652353));
#64294=CARTESIAN_POINT('Ctrl Pts',(26.5,18.5112642482312,-20.3428774672885));
#64295=CARTESIAN_POINT('Ctrl Pts',(26.5,19.0613782547939,-19.8237187585295));
#64296=CARTESIAN_POINT('Ctrl Pts',(26.4810497169031,19.2549528183989,-19.6359201468613));
#64297=CARTESIAN_POINT('Ctrl Pts',(26.4377160017535,19.4454364826275,-19.4454364826326));
#64298=CARTESIAN_POINT('',(26.7834228088254,12.,24.7436860633173));
#64299=CARTESIAN_POINT('',(21.2165771911746,12.,24.7436860633173));
#64300=CARTESIAN_POINT('',(24.,12.,24.7436860633173));
#64301=CARTESIAN_POINT('Ctrl Pts',(21.2165771911746,12.,24.7436860633173));
#64302=CARTESIAN_POINT('Ctrl Pts',(20.9800185926029,12.2862102160665,24.6048820636218));
#64303=CARTESIAN_POINT('Ctrl Pts',(20.764413790233,12.5833300005747,24.4543921279647));
#64304=CARTESIAN_POINT('Ctrl Pts',(19.9481928010976,13.811462707463,23.8038074123085));
#64305=CARTESIAN_POINT('Ctrl Pts',(19.4277281498764,14.8735636803617,23.1658933876871));
#64306=CARTESIAN_POINT('Ctrl Pts',(18.7008421968431,16.9568964437325,21.6874432584144));
#64307=CARTESIAN_POINT('Ctrl Pts',(18.5,17.9789117753936,20.8452740961799));
#64308=CARTESIAN_POINT('Ctrl Pts',(18.5,19.5518661056715,19.3608310001999));
#64309=CARTESIAN_POINT('Ctrl Pts',(18.6175304465914,20.2511953036901,18.6288115221753));
#64310=CARTESIAN_POINT('Ctrl Pts',(19.2063453548323,21.4825503875294,17.1942881563934));
#64311=CARTESIAN_POINT('Ctrl Pts',(19.680056660858,22.0156394470847,16.4936948503358));
#64312=CARTESIAN_POINT('Ctrl Pts',(20.7520277927281,22.707492236193,15.5200247473001));
#64313=CARTESIAN_POINT('Ctrl Pts',(21.3285452412578,22.9573233129958,15.1427702692175));
#64314=CARTESIAN_POINT('Ctrl Pts',(22.6156966073876,23.2860541564014,14.6322199108483));
#64315=CARTESIAN_POINT('Ctrl Pts',(23.3263251783664,23.3666428910959,14.5));
#64316=CARTESIAN_POINT('Ctrl Pts',(24.6736748216336,23.3666428910959,14.5));
#64317=CARTESIAN_POINT('Ctrl Pts',(25.3843033926124,23.2860541564014,14.6322199108483));
#64318=CARTESIAN_POINT('Ctrl Pts',(26.6714547587422,22.9573233129958,15.1427702692175));
#64319=CARTESIAN_POINT('Ctrl Pts',(27.2479722072719,22.707492236193,15.5200247473001));
#64320=CARTESIAN_POINT('Ctrl Pts',(28.319943339142,22.0156394470847,16.4936948503358));
#64321=CARTESIAN_POINT('Ctrl Pts',(28.7936546451677,21.4825503875294,17.1942881563934));
#64322=CARTESIAN_POINT('Ctrl Pts',(29.3824695534086,20.2511953036901,18.6288115221753));
#64323=CARTESIAN_POINT('Ctrl Pts',(29.5,19.5518661056715,19.3608310001999));
#64324=CARTESIAN_POINT('Ctrl Pts',(29.5,17.9789117753936,20.8452740961799));
#64325=CARTESIAN_POINT('Ctrl Pts',(29.2991578031569,16.9568964437325,21.6874432584144));
#64326=CARTESIAN_POINT('Ctrl Pts',(28.5722718501237,14.8735636803618,23.1658933876871));
#64327=CARTESIAN_POINT('Ctrl Pts',(28.0518071989025,13.811462707463,23.8038074123085));
#64328=CARTESIAN_POINT('Ctrl Pts',(27.235586209767,12.5833300005747,24.4543921279647));
#64329=CARTESIAN_POINT('Ctrl Pts',(27.0199814073971,12.2862102160665,24.6048820636218));
#64330=CARTESIAN_POINT('Ctrl Pts',(26.7834228088254,12.,24.7436860633173));
#64331=CARTESIAN_POINT('Origin',(24.,0.,0.));
#64332=CARTESIAN_POINT('',(9.,0.1,5.99916660878826));
#64333=CARTESIAN_POINT('',(24.,0.1,5.99916660878826));
#64334=CARTESIAN_POINT('',(9.,0.1,-5.99916660878826));
#64335=CARTESIAN_POINT('Origin',(9.,0.,0.));
#64336=CARTESIAN_POINT('',(24.,0.1,-5.99916660878826));
#64337=CARTESIAN_POINT('Origin',(9.,0.,-22.5));
#64338=CARTESIAN_POINT('',(9.,0.1,-11.25));
#64339=CARTESIAN_POINT('',(9.,0.1,-11.25));
#64340=CARTESIAN_POINT('Origin',(24.,12.25,-20.));
#64341=CARTESIAN_POINT('',(21.5,0.1,-20.));
#64342=CARTESIAN_POINT('',(21.5,12.25,-20.));
#64343=CARTESIAN_POINT('Origin',(24.,0.1,-20.));
#64344=CARTESIAN_POINT('Origin',(28.4,12.,20.));
#64345=CARTESIAN_POINT('Origin',(24.,12.,20.));
#64346=CARTESIAN_POINT('',(20.7,12.,20.));
#64347=CARTESIAN_POINT('Origin',(24.,12.,20.));
#64348=CARTESIAN_POINT('Origin',(24.,7.5,20.));
#64349=CARTESIAN_POINT('',(20.7,3.,20.));
#64350=CARTESIAN_POINT('Origin',(24.,3.,20.));
#64351=CARTESIAN_POINT('',(20.7,7.5,20.));
#64352=CARTESIAN_POINT('Origin',(26.9,3.,20.));
#64353=CARTESIAN_POINT('',(21.5,3.,20.));
#64354=CARTESIAN_POINT('Origin',(24.,3.,20.));
#64355=CARTESIAN_POINT('Origin',(24.,-12.25,20.));
#64356=CARTESIAN_POINT('',(21.5,0.1,20.));
#64357=CARTESIAN_POINT('Origin',(24.,0.1,20.));
#64358=CARTESIAN_POINT('',(21.5,-12.25,20.));
#64359=CARTESIAN_POINT('Origin',(16.,0.1,0.));
#64360=CARTESIAN_POINT('Origin',(16.,0.1,0.));
#64361=CARTESIAN_POINT('Origin',(24.,19.75,20.));
#64362=CARTESIAN_POINT('Origin',(24.,-19.75,-20.));
#64363=CARTESIAN_POINT('',(26.7834228088254,-12.,-24.7436860633173));
#64364=CARTESIAN_POINT('',(21.2165771911746,-12.,-24.7436860633173));
#64365=CARTESIAN_POINT('Origin',(24.,-12.,-20.));
#64366=CARTESIAN_POINT('Ctrl Pts',(26.7834228088254,-12.,-24.7436860633173));
#64367=CARTESIAN_POINT('Ctrl Pts',(27.019981407397,-12.2862102160664,-24.6048820636218));
#64368=CARTESIAN_POINT('Ctrl Pts',(27.235586209767,-12.5833300005747,-24.4543921279647));
#64369=CARTESIAN_POINT('Ctrl Pts',(28.0518071989025,-13.811462707463,-23.8038074123085));
#64370=CARTESIAN_POINT('Ctrl Pts',(28.5722718501237,-14.8735636803618,-23.1658933876871));
#64371=CARTESIAN_POINT('Ctrl Pts',(29.2991578031569,-16.9568964437325,-21.6874432584144));
#64372=CARTESIAN_POINT('Ctrl Pts',(29.5,-17.9789117753936,-20.8452740961799));
#64373=CARTESIAN_POINT('Ctrl Pts',(29.5,-19.5518661056715,-19.3608310001999));
#64374=CARTESIAN_POINT('Ctrl Pts',(29.3824695534086,-20.2511953036901,-18.6288115221753));
#64375=CARTESIAN_POINT('Ctrl Pts',(28.7936546451677,-21.4825503875294,-17.1942881563934));
#64376=CARTESIAN_POINT('Ctrl Pts',(28.319943339142,-22.0156394470847,-16.4936948503358));
#64377=CARTESIAN_POINT('Ctrl Pts',(27.2479722072719,-22.707492236193,-15.5200247473001));
#64378=CARTESIAN_POINT('Ctrl Pts',(26.6714547587422,-22.9573233129958,-15.1427702692175));
#64379=CARTESIAN_POINT('Ctrl Pts',(25.3843033926124,-23.2860541564014,-14.6322199108483));
#64380=CARTESIAN_POINT('Ctrl Pts',(24.6736748216336,-23.3666428910959,-14.5));
#64381=CARTESIAN_POINT('Ctrl Pts',(23.3263251783664,-23.3666428910959,-14.5));
#64382=CARTESIAN_POINT('Ctrl Pts',(22.6156966073876,-23.2860541564014,-14.6322199108483));
#64383=CARTESIAN_POINT('Ctrl Pts',(21.3285452412578,-22.9573233129958,-15.1427702692175));
#64384=CARTESIAN_POINT('Ctrl Pts',(20.7520277927281,-22.707492236193,-15.5200247473001));
#64385=CARTESIAN_POINT('Ctrl Pts',(19.680056660858,-22.0156394470847,-16.4936948503358));
#64386=CARTESIAN_POINT('Ctrl Pts',(19.2063453548323,-21.4825503875294,-17.1942881563934));
#64387=CARTESIAN_POINT('Ctrl Pts',(18.6175304465914,-20.2511953036901,-18.6288115221753));
#64388=CARTESIAN_POINT('Ctrl Pts',(18.5,-19.5518661056715,-19.3608310001999));
#64389=CARTESIAN_POINT('Ctrl Pts',(18.5,-17.9789117753936,-20.8452740961799));
#64390=CARTESIAN_POINT('Ctrl Pts',(18.7008421968431,-16.9568964437325,-21.6874432584144));
#64391=CARTESIAN_POINT('Ctrl Pts',(19.4277281498764,-14.8735636803617,-23.1658933876871));
#64392=CARTESIAN_POINT('Ctrl Pts',(19.9481928010976,-13.811462707463,-23.8038074123085));
#64393=CARTESIAN_POINT('Ctrl Pts',(20.764413790233,-12.5833300005747,-24.4543921279647));
#64394=CARTESIAN_POINT('Ctrl Pts',(20.980018592603,-12.2862102160665,-24.6048820636218));
#64395=CARTESIAN_POINT('Ctrl Pts',(21.2165771911746,-12.,-24.7436860633173));
#64396=CARTESIAN_POINT('Origin',(16.,-0.1,0.));
#64397=CARTESIAN_POINT('',(39.,-0.1,25.9998076915965));
#64398=CARTESIAN_POINT('',(37.5,-0.1,27.4998181812171));
#64399=CARTESIAN_POINT('',(38.25,-0.1,26.7498129364068));
#64400=CARTESIAN_POINT('',(39.,-0.1,5.99916660878826));
#64401=CARTESIAN_POINT('',(39.,-0.1,4.59619407771256));
#64402=CARTESIAN_POINT('',(9.,-0.1,5.99916660878826));
#64403=CARTESIAN_POINT('',(24.,-0.1,5.99916660878826));
#64404=CARTESIAN_POINT('',(9.,-0.1,27.4998181812171));
#64405=CARTESIAN_POINT('',(9.,-0.1,-11.25));
#64406=CARTESIAN_POINT('',(15.25,-0.1,27.4998181812171));
#64407=CARTESIAN_POINT('',(21.5,-0.1,20.));
#64408=CARTESIAN_POINT('Origin',(24.,-0.1,20.));
#64409=CARTESIAN_POINT('Origin',(24.,-12.25,20.));
#64410=CARTESIAN_POINT('',(24.,-15.8113883008419,22.5));
#64411=CARTESIAN_POINT('',(21.5,-18.8745860881769,20.));
#64412=CARTESIAN_POINT('Ctrl Pts',(21.5,-18.8745860881769,20.));
#64413=CARTESIAN_POINT('Ctrl Pts',(21.5,-19.1981343317555,19.6946580411449));
#64414=CARTESIAN_POINT('Ctrl Pts',(21.5586819382302,-19.5412928441449,19.3544362091167));
#64415=CARTESIAN_POINT('Ctrl Pts',(21.8359982780239,-20.169832853608,18.6985071174812));
#64416=CARTESIAN_POINT('Ctrl Pts',(22.054836947176,-20.4554595320486,18.383121240662));
#64417=CARTESIAN_POINT('Ctrl Pts',(22.5416783856535,-20.8332972173375,17.9521176633326));
#64418=CARTESIAN_POINT('Ctrl Pts',(22.7968722688251,-20.9737985255456,17.7868382119765));
#64419=CARTESIAN_POINT('Ctrl Pts',(23.3723171754151,-21.1637417254346,17.5604063991252));
#64420=CARTESIAN_POINT('Ctrl Pts',(23.6928549082306,-21.2132034355965,17.5));
#64421=CARTESIAN_POINT('Ctrl Pts',(24.3071450917694,-21.2132034355965,17.5));
#64422=CARTESIAN_POINT('Ctrl Pts',(24.627682824585,-21.1637417254346,17.5604063991252));
#64423=CARTESIAN_POINT('Ctrl Pts',(25.2031277311749,-20.9737985255456,17.7868382119765));
#64424=CARTESIAN_POINT('Ctrl Pts',(25.4583216143465,-20.8332972173375,17.9521176633326));
#64425=CARTESIAN_POINT('Ctrl Pts',(25.945163052824,-20.4554595320486,18.383121240662));
#64426=CARTESIAN_POINT('Ctrl Pts',(26.1640017219762,-20.169832853608,18.6985071174812));
#64427=CARTESIAN_POINT('Ctrl Pts',(26.4413180617698,-19.5412928441449,19.3544362091167));
#64428=CARTESIAN_POINT('Ctrl Pts',(26.5,-19.1981343317555,19.6946580411449));
#64429=CARTESIAN_POINT('Ctrl Pts',(26.5,-18.5112642482312,20.3428774672885));
#64430=CARTESIAN_POINT('Ctrl Pts',(26.4267189640483,-18.1082220917789,20.7028459652353));
#64431=CARTESIAN_POINT('Ctrl Pts',(26.1248673898206,-17.3199088998874,21.3667099444405));
#64432=CARTESIAN_POINT('Ctrl Pts',(25.8980213172189,-16.9344413423488,21.6711549104462));
#64433=CARTESIAN_POINT('Ctrl Pts',(25.4199810017124,-16.4058021284168,22.0718427713117));
#64434=CARTESIAN_POINT('Ctrl Pts',(25.1823324639043,-16.2001944002355,22.222452745926));
#64435=CARTESIAN_POINT('Ctrl Pts',(24.7695622900288,-15.976589433265,22.3831860081774));
#64436=CARTESIAN_POINT('Ctrl Pts',(24.6225767382908,-15.9159206638649,22.4262333390977));
#64437=CARTESIAN_POINT('Ctrl Pts',(24.3173127716233,-15.8333169759962,22.4846329655715));
#64438=CARTESIAN_POINT('Ctrl Pts',(24.1590354871529,-15.8113883008419,22.5));
#64439=CARTESIAN_POINT('Ctrl Pts',(24.,-15.8113883008419,22.5));
#64440=CARTESIAN_POINT('Ctrl Pts',(24.,-15.8113883008419,22.5));
#64441=CARTESIAN_POINT('Ctrl Pts',(23.8409645128471,-15.8113883008419,22.5));
#64442=CARTESIAN_POINT('Ctrl Pts',(23.6826872283767,-15.8333169759962,22.4846329655715));
#64443=CARTESIAN_POINT('Ctrl Pts',(23.3774232617092,-15.9159206638649,22.4262333390977));
#64444=CARTESIAN_POINT('Ctrl Pts',(23.2304377099712,-15.976589433265,22.3831860081774));
#64445=CARTESIAN_POINT('Ctrl Pts',(22.8176675360957,-16.2001944002355,22.222452745926));
#64446=CARTESIAN_POINT('Ctrl Pts',(22.5800189982876,-16.4058021284168,22.0718427713117));
#64447=CARTESIAN_POINT('Ctrl Pts',(22.1019786827811,-16.9344413423488,21.6711549104462));
#64448=CARTESIAN_POINT('Ctrl Pts',(21.8751326101794,-17.3199088998874,21.3667099444405));
#64449=CARTESIAN_POINT('Ctrl Pts',(21.5732810359517,-18.1082220917789,20.7028459652353));
#64450=CARTESIAN_POINT('Ctrl Pts',(21.5,-18.5112642482312,20.3428774672885));
#64451=CARTESIAN_POINT('Ctrl Pts',(21.5,-18.8745860881769,20.));
#64452=CARTESIAN_POINT('',(21.5,-12.25,20.));
#64453=CARTESIAN_POINT('Origin',(24.,12.25,-20.));
#64454=CARTESIAN_POINT('',(21.5,-0.1,-20.));
#64455=CARTESIAN_POINT('Origin',(24.,-0.1,-20.));
#64456=CARTESIAN_POINT('',(21.5,-3.,-20.));
#64457=CARTESIAN_POINT('',(21.5,12.25,-20.));
#64458=CARTESIAN_POINT('Origin',(24.,-3.,-20.));
#64459=CARTESIAN_POINT('Origin',(26.9,-3.,-20.));
#64460=CARTESIAN_POINT('',(20.7,-3.,-20.));
#64461=CARTESIAN_POINT('Origin',(24.,-3.,-20.));
#64462=CARTESIAN_POINT('Origin',(24.,-7.5,-20.));
#64463=CARTESIAN_POINT('',(20.7,-12.,-20.));
#64464=CARTESIAN_POINT('',(20.7,-7.5,-20.));
#64465=CARTESIAN_POINT('Origin',(24.,-12.,-20.));
#64466=CARTESIAN_POINT('Origin',(28.4,-12.,-20.));
#64467=CARTESIAN_POINT('',(24.,-12.,-24.7436860633173));
#64468=CARTESIAN_POINT('Origin',(16.,-0.1,0.));
#64469=CARTESIAN_POINT('',(37.5,-0.1,-27.4998181812171));
#64470=CARTESIAN_POINT('',(39.,-0.1,-25.9998076915965));
#64471=CARTESIAN_POINT('',(38.25,-0.1,-26.7498129364068));
#64472=CARTESIAN_POINT('',(9.,-0.1,-27.4998181812171));
#64473=CARTESIAN_POINT('',(15.25,-0.1,-27.4998181812171));
#64474=CARTESIAN_POINT('',(9.,-0.1,-5.99916660878826));
#64475=CARTESIAN_POINT('',(9.,-0.1,-11.25));
#64476=CARTESIAN_POINT('',(39.,-0.1,-5.99916660878826));
#64477=CARTESIAN_POINT('',(24.,-0.1,-5.99916660878826));
#64478=CARTESIAN_POINT('',(39.,-0.1,4.59619407771256));
#64479=CARTESIAN_POINT('Origin',(39.,-9.19238815542512,9.19238815542512));
#64480=CARTESIAN_POINT('',(39.,-5.65685424949238,-2.));
#64481=CARTESIAN_POINT('Origin',(39.,0.,0.));
#64482=CARTESIAN_POINT('',(39.,-7.8,-2.));
#64483=CARTESIAN_POINT('',(39.,-6.54619407771256,-2.));
#64484=CARTESIAN_POINT('',(39.,-7.8,2.));
#64485=CARTESIAN_POINT('',(39.,-7.8,4.59619407771256));
#64486=CARTESIAN_POINT('',(39.,-5.65685424949238,2.));
#64487=CARTESIAN_POINT('',(39.,-6.54619407771256,2.));
#64488=CARTESIAN_POINT('Origin',(39.,0.,0.));
#64489=CARTESIAN_POINT('Origin',(39.,0.,0.));
#64490=CARTESIAN_POINT('Origin',(38.25,0.,0.));
#64491=CARTESIAN_POINT('Origin',(37.5,0.,0.));
#64492=CARTESIAN_POINT('Origin',(9.,0.,-22.5));
#64493=CARTESIAN_POINT('',(9.,-12.8747815515449,-24.3));
#64494=CARTESIAN_POINT('Origin',(9.,0.,0.));
#64495=CARTESIAN_POINT('',(9.,-10.0876161703348,-14.3));
#64496=CARTESIAN_POINT('Origin',(9.,0.,-22.5));
#64497=CARTESIAN_POINT('',(9.,-14.3,-10.0876161703348));
#64498=CARTESIAN_POINT('Origin',(9.,0.,0.));
#64499=CARTESIAN_POINT('',(9.,-24.3,-12.8747815515449));
#64500=CARTESIAN_POINT('Origin',(9.,-22.5,0.));
#64501=CARTESIAN_POINT('',(9.,-24.3,12.8747815515449));
#64502=CARTESIAN_POINT('Origin',(9.,0.,0.));
#64503=CARTESIAN_POINT('',(9.,-14.3,10.0876161703348));
#64504=CARTESIAN_POINT('Origin',(9.,-22.5,0.));
#64505=CARTESIAN_POINT('',(9.,-10.0876161703348,14.3));
#64506=CARTESIAN_POINT('Origin',(9.,0.,0.));
#64507=CARTESIAN_POINT('',(9.,-12.8747815515449,24.3));
#64508=CARTESIAN_POINT('Origin',(9.,0.,22.5));
#64509=CARTESIAN_POINT('Origin',(9.,0.,0.));
#64510=CARTESIAN_POINT('',(9.,-5.65685424949238,2.));
#64511=CARTESIAN_POINT('Origin',(9.,0.,0.));
#64512=CARTESIAN_POINT('',(9.,-7.8,2.));
#64513=CARTESIAN_POINT('',(9.,-1.95,2.));
#64514=CARTESIAN_POINT('',(9.,-7.8,-2.));
#64515=CARTESIAN_POINT('',(9.,-7.8,-11.25));
#64516=CARTESIAN_POINT('',(9.,-5.65685424949238,-2.));
#64517=CARTESIAN_POINT('',(9.,-1.95,-2.));
#64518=CARTESIAN_POINT('Origin',(9.,0.,0.));
#64519=CARTESIAN_POINT('Origin',(24.,0.,0.));
#64520=CARTESIAN_POINT('',(29.6403124237433,-5.65685424949238,2.));
#64521=CARTESIAN_POINT('',(24.,-5.65685424949238,2.));
#64522=CARTESIAN_POINT('',(28.3596875762567,-5.65685424949238,2.));
#64523=CARTESIAN_POINT('Ctrl Pts',(28.3596875762567,-5.65685424949239,1.99999999999999));
#64524=CARTESIAN_POINT('Ctrl Pts',(28.5698259640486,-5.63306819907035,2.06727711020427));
#64525=CARTESIAN_POINT('Ctrl Pts',(28.7900272337845,-5.62049819855856,2.1));
#64526=CARTESIAN_POINT('Ctrl Pts',(29.2099727662155,-5.62049819855856,2.1));
#64527=CARTESIAN_POINT('Ctrl Pts',(29.4301740359514,-5.63306819907034,2.06727711020428));
#64528=CARTESIAN_POINT('Ctrl Pts',(29.6403124237433,-5.65685424949239,2.));
#64529=CARTESIAN_POINT('',(24.,-5.65685424949238,2.));
#64530=CARTESIAN_POINT('Origin',(24.,0.,0.));
#64531=CARTESIAN_POINT('',(28.3596875762567,-5.65685424949238,-2.));
#64532=CARTESIAN_POINT('',(24.,-5.65685424949238,-2.));
#64533=CARTESIAN_POINT('',(29.6403124237433,-5.65685424949238,-2.));
#64534=CARTESIAN_POINT('Ctrl Pts',(29.6403124237433,-5.65685424949239,-2.));
#64535=CARTESIAN_POINT('Ctrl Pts',(29.4301740359514,-5.63306819907035,-2.06727711020427));
#64536=CARTESIAN_POINT('Ctrl Pts',(29.2099727662155,-5.62049819855856,-2.1));
#64537=CARTESIAN_POINT('Ctrl Pts',(29.,-5.62049819855856,-2.1));
#64538=CARTESIAN_POINT('Ctrl Pts',(28.7900272337845,-5.62049819855856,-2.1));
#64539=CARTESIAN_POINT('Ctrl Pts',(28.5698259640486,-5.63306819907035,-2.06727711020427));
#64540=CARTESIAN_POINT('Ctrl Pts',(28.3596875762567,-5.65685424949239,-2.));
#64541=CARTESIAN_POINT('',(24.,-5.65685424949238,-2.));
#64542=CARTESIAN_POINT('Origin',(15.25,0.,0.));
#64543=CARTESIAN_POINT('',(3.7202200813,-19.2325444488655,19.6560228434547));
#64544=CARTESIAN_POINT('',(4.3435534146,-19.2325444488655,19.6560228434547));
#64545=CARTESIAN_POINT('',(4.03188674795,-19.2325444488655,19.6560228434547));
#64546=CARTESIAN_POINT('',(4.3435534146,-18.6475617704547,20.2118391052639));
#64547=CARTESIAN_POINT('Ctrl Pts',(4.3435534146,-19.2325444488655,19.6560228434547));
#64548=CARTESIAN_POINT('Ctrl Pts',(4.39419602744118,-19.2325444488655,19.6560228434547));
#64549=CARTESIAN_POINT('Ctrl Pts',(4.44821405117923,-19.2253141398743,19.6631055485021));
#64550=CARTESIAN_POINT('Ctrl Pts',(4.54758440972013,-19.1958605065015,19.6918603235793));
#64551=CARTESIAN_POINT('Ctrl Pts',(4.59293670765284,-19.1736315324598,19.7135267334984));
#64552=CARTESIAN_POINT('Ctrl Pts',(4.66456223528332,-19.1222183158652,19.7634017741075));
#64553=CARTESIAN_POINT('Ctrl Pts',(4.69560557365306,-19.0896044189134,19.7949355413725));
#64554=CARTESIAN_POINT('Ctrl Pts',(4.7367677324877,-19.0179321794404,19.8638044084183));
#64555=CARTESIAN_POINT('Ctrl Pts',(4.7468867479,-18.9788683526504,19.9011336839378));
#64556=CARTESIAN_POINT('Ctrl Pts',(4.7468867479,-18.9054144267782,19.9709256846039));
#64557=CARTESIAN_POINT('Ctrl Pts',(4.73676246101481,-18.8661272497408,20.0080412374082));
#64558=CARTESIAN_POINT('Ctrl Pts',(4.69559144465381,-18.7936626617373,20.0761230151159));
#64559=CARTESIAN_POINT('Ctrl Pts',(4.66454479714166,-18.7604907000729,20.1070950894545));
#64560=CARTESIAN_POINT('Ctrl Pts',(4.59292152712871,-18.7080352594837,20.1559097961516));
#64561=CARTESIAN_POINT('Ctrl Pts',(4.54757596140155,-18.6852506642774,20.1770124569941));
#64562=CARTESIAN_POINT('Ctrl Pts',(4.44821406584017,-18.6550109864893,20.2049743669883));
#64563=CARTESIAN_POINT('Ctrl Pts',(4.39419749547155,-18.6475617704547,20.2118391052639));
#64564=CARTESIAN_POINT('Ctrl Pts',(4.3435534146,-18.6475617704547,20.2118391052639));
#64565=CARTESIAN_POINT('',(3.7202200813,-18.6475617704547,20.2118391052639));
#64566=CARTESIAN_POINT('',(4.03188674795,-18.6475617704547,20.2118391052639));
#64567=CARTESIAN_POINT('Origin',(3.7202200813,0.,0.));
#64568=CARTESIAN_POINT('Origin',(29.,-13.75,0.));
#64569=CARTESIAN_POINT('',(29.6403124237433,-7.8,2.));
#64570=CARTESIAN_POINT('',(31.1,-7.8,2.57175827820944E-16));
#64571=CARTESIAN_POINT('Origin',(29.,-7.8,0.));
#64572=CARTESIAN_POINT('',(31.1,-27.5,2.57175827820944E-16));
#64573=CARTESIAN_POINT('',(31.1,-13.75,2.57175827820944E-16));
#64574=CARTESIAN_POINT('',(26.9,-27.5,0.));
#64575=CARTESIAN_POINT('Ctrl Pts',(26.9,-27.5,-4.16333634234434E-16));
#64576=CARTESIAN_POINT('Ctrl Pts',(26.9,-27.5,0.263790724669232));
#64577=CARTESIAN_POINT('Ctrl Pts',(26.9527396524836,-27.4958150675353,0.5450944837367));
#64578=CARTESIAN_POINT('Ctrl Pts',(27.167084371912,-27.4806868728543,1.06246092692353));
#64579=CARTESIAN_POINT('Ctrl Pts',(27.3286837627136,-27.4699591842076,1.29853224369707));
#64580=CARTESIAN_POINT('Ctrl Pts',(27.7014679712018,-27.4498004540462,1.67131645218531));
#64581=CARTESIAN_POINT('Ctrl Pts',(27.9375391926626,-27.4390590848186,1.83291567693009));
#64582=CARTESIAN_POINT('Ctrl Pts',(28.4549053217882,-27.423899590768,2.04726026764777));
#64583=CARTESIAN_POINT('Ctrl Pts',(28.7362089711958,-27.4197009465822,2.1));
#64584=CARTESIAN_POINT('Ctrl Pts',(29.2637910288042,-27.4197009465822,2.1));
#64585=CARTESIAN_POINT('Ctrl Pts',(29.5450946782118,-27.423899590768,2.04726026764777));
#64586=CARTESIAN_POINT('Ctrl Pts',(30.0624608073374,-27.4390590848186,1.8329156769301));
#64587=CARTESIAN_POINT('Ctrl Pts',(30.2985320287982,-27.4498004540462,1.67131645218531));
#64588=CARTESIAN_POINT('Ctrl Pts',(30.6713162372864,-27.4699591842076,1.29853224369707));
#64589=CARTESIAN_POINT('Ctrl Pts',(30.832915628088,-27.4806868728543,1.06246092692352));
#64590=CARTESIAN_POINT('Ctrl Pts',(31.0472603475164,-27.4958150675353,0.545094483736699));
#64591=CARTESIAN_POINT('Ctrl Pts',(31.1,-27.5,0.263790724669232));
#64592=CARTESIAN_POINT('Ctrl Pts',(31.1,-27.5,-4.85722573273506E-16));
#64593=CARTESIAN_POINT('',(29.,-27.4197009465822,-2.1));
#64594=CARTESIAN_POINT('Ctrl Pts',(29.,-27.4197009465822,-2.1));
#64595=CARTESIAN_POINT('Ctrl Pts',(28.9409243313237,-27.4197009465822,-2.1));
#64596=CARTESIAN_POINT('Ctrl Pts',(28.8823185718112,-27.41989199691,-2.09751141842624));
#64597=CARTESIAN_POINT('Ctrl Pts',(28.8241875421993,-27.4202649703079,-2.09262753008797));
#64598=CARTESIAN_POINT('Ctrl Pts',(28.7651735223191,-27.4206436090429,-2.08766945717214));
#64599=CARTESIAN_POINT('Ctrl Pts',(28.7066479007282,-27.4212097395195,-2.08024281822867));
#64600=CARTESIAN_POINT('Ctrl Pts',(28.6486082408746,-27.4219538122106,-2.07039219270619));
#64601=CARTESIAN_POINT('Ctrl Pts',(28.5905518712427,-27.4226980991222,-2.06053873116144));
#64602=CARTESIAN_POINT('Ctrl Pts',(28.532980875708,-27.4236204307232,-2.04825974278311));
#64603=CARTESIAN_POINT('Ctrl Pts',(28.4758984634574,-27.424711249236,-2.03354802731425));
#64604=CARTESIAN_POINT('Ctrl Pts',(28.4194214360888,-27.4257904991236,-2.01899233626311));
#64605=CARTESIAN_POINT('Ctrl Pts',(28.3634218905768,-27.4270346811134,-2.00205494714711));
#64606=CARTESIAN_POINT('Ctrl Pts',(28.3079207704063,-27.4284345383079,-1.98268160327497));
#64607=CARTESIAN_POINT('Ctrl Pts',(28.2704559711509,-27.4293794808355,-1.96960405750932));
#64608=CARTESIAN_POINT('Ctrl Pts',(28.2332186617402,-27.4303953587217,-1.95541555925643));
#64609=CARTESIAN_POINT('Ctrl Pts',(28.1962227045941,-27.4314793246848,-1.94008815763357));
#64610=CARTESIAN_POINT('Ctrl Pts',(28.1419909448439,-27.4330682924051,-1.91761997390408));
#64611=CARTESIAN_POINT('Ctrl Pts',(28.0891325285996,-27.434776870226,-1.89306111287472));
#64612=CARTESIAN_POINT('Ctrl Pts',(28.0376128725783,-27.4365837911004,-1.8664969908824));
#64613=CARTESIAN_POINT('Ctrl Pts',(27.9853278197182,-27.4384175563217,-1.83953822155411));
#64614=CARTESIAN_POINT('Ctrl Pts',(27.9344207893789,-27.4403526083505,-1.81051389260381));
#64615=CARTESIAN_POINT('Ctrl Pts',(27.8848692034387,-27.4423667181325,-1.77946152151725));
#64616=CARTESIAN_POINT('Ctrl Pts',(27.8353096468437,-27.4443811518955,-1.74840415547999));
#64617=CARTESIAN_POINT('Ctrl Pts',(27.787105233271,-27.4464746688476,-1.71531763408417));
#64618=CARTESIAN_POINT('Ctrl Pts',(27.7402584733154,-27.448625029206,-1.6801938239222));
#64619=CARTESIAN_POINT('Ctrl Pts',(27.6939156420422,-27.4507522582258,-1.6454478391508));
#64620=CARTESIAN_POINT('Ctrl Pts',(27.6489008015155,-27.452935114305,-1.60870758824503));
#64621=CARTESIAN_POINT('Ctrl Pts',(27.6052508774519,-27.4551520676655,-1.56992830573606));
#64622=CARTESIAN_POINT('Ctrl Pts',(27.5745062828372,-27.4567135671138,-1.54261432190297));
#64623=CARTESIAN_POINT('Ctrl Pts',(27.5444395290512,-27.4582919822752,-1.51428798453775));
#64624=CARTESIAN_POINT('Ctrl Pts',(27.515076404205,-27.4598797900746,-1.48492488518827));
#64625=CARTESIAN_POINT('Ctrl Pts',(27.4739307804,-27.4621047352306,-1.44377929711088));
#64626=CARTESIAN_POINT('Ctrl Pts',(27.4348258111026,-27.464310388427,-1.40126006169301));
#64627=CARTESIAN_POINT('Ctrl Pts',(27.3976932514178,-27.4664763150051,-1.35742885023417));
#64628=CARTESIAN_POINT('Ctrl Pts',(27.3600131664037,-27.4686741785051,-1.31295134079059));
#64629=CARTESIAN_POINT('Ctrl Pts',(27.324363452127,-27.4708311351993,-1.26712232282476));
#64630=CARTESIAN_POINT('Ctrl Pts',(27.2907051879064,-27.472925833098,-1.21996362460113));
#64631=CARTESIAN_POINT('Ctrl Pts',(27.2570404827003,-27.4750209318468,-1.17279590189273));
#64632=CARTESIAN_POINT('Ctrl Pts',(27.2253674916476,-27.4770537479697,-1.12429729314642));
#64633=CARTESIAN_POINT('Ctrl Pts',(27.1956878552808,-27.4790029172168,-1.07445692534351));
#64634=CARTESIAN_POINT('Ctrl Pts',(27.1663254278886,-27.4809312542013,-1.02514923967236));
#64635=CARTESIAN_POINT('Ctrl Pts',(27.1389136304772,-27.4827777227514,-0.974527572618045));
#64636=CARTESIAN_POINT('Ctrl Pts',(27.1134998926964,-27.4845216363304,-0.922560212204816));
#64637=CARTESIAN_POINT('Ctrl Pts',(27.0945077136406,-27.4858248967652,-0.883723996039469));
#64638=CARTESIAN_POINT('Ctrl Pts',(27.0766323337252,-27.4870708816564,-0.84413572170515));
#64639=CARTESIAN_POINT('Ctrl Pts',(27.0599121975429,-27.4882509571134,-0.803778152699582));
#64640=CARTESIAN_POINT('Ctrl Pts',(27.0375591557555,-27.4898285923499,-0.749824380039959));
#64641=CARTESIAN_POINT('Ctrl Pts',(27.0176337763087,-27.4912611977169,-0.695376406081773));
#64642=CARTESIAN_POINT('Ctrl Pts',(27.0000496507938,-27.4925402285157,-0.640467486067715));
#64643=CARTESIAN_POINT('Ctrl Pts',(26.9822027462824,-27.4938383732835,-0.584738001454926));
#64644=CARTESIAN_POINT('Ctrl Pts',(26.9667672171644,-27.4949783191173,-0.52853293039682));
#64645=CARTESIAN_POINT('Ctrl Pts',(26.9536989008167,-27.4959511324866,-0.47185994901157));
#64646=CARTESIAN_POINT('Ctrl Pts',(26.9406270335015,-27.496924210192,-0.415171568250305));
#64647=CARTESIAN_POINT('Ctrl Pts',(26.9299234702452,-27.4977300645931,-0.358014183201836));
#64648=CARTESIAN_POINT('Ctrl Pts',(26.9215940204666,-27.4983597548748,-0.30038073213773));
#64649=CARTESIAN_POINT('Ctrl Pts',(26.9133527431796,-27.4989827794868,-0.243357367588823));
#64650=CARTESIAN_POINT('Ctrl Pts',(26.9074355517769,-27.4994333498565,-0.185867132809557));
#64651=CARTESIAN_POINT('Ctrl Pts',(26.9038985506734,-27.4997028061065,-0.127901188933921));
#64652=CARTESIAN_POINT('Ctrl Pts',(26.9013126263583,-27.4998998073085,-0.0855219135745074));
#64653=CARTESIAN_POINT('Ctrl Pts',(26.9,-27.5,-0.0428882664061002));
#64654=CARTESIAN_POINT('Ctrl Pts',(26.9,-27.5,0.));
#64655=CARTESIAN_POINT('Ctrl Pts',(31.1,-27.5,-3.46944695195361E-16));
#64656=CARTESIAN_POINT('Ctrl Pts',(31.1,-27.5,-0.263790724669233));
#64657=CARTESIAN_POINT('Ctrl Pts',(31.0472603475164,-27.4958150675353,-0.545094483736701));
#64658=CARTESIAN_POINT('Ctrl Pts',(30.832915628088,-27.4806868728543,-1.06246092692353));
#64659=CARTESIAN_POINT('Ctrl Pts',(30.6713162372864,-27.4699591842076,-1.29853224369707));
#64660=CARTESIAN_POINT('Ctrl Pts',(30.2985320287982,-27.4498004540462,-1.67131645218531));
#64661=CARTESIAN_POINT('Ctrl Pts',(30.0624608073374,-27.4390590848186,-1.8329156769301));
#64662=CARTESIAN_POINT('Ctrl Pts',(29.5450946782118,-27.423899590768,-2.04726026764777));
#64663=CARTESIAN_POINT('Ctrl Pts',(29.2637910288042,-27.4197009465822,-2.1));
#64664=CARTESIAN_POINT('Ctrl Pts',(29.,-27.4197009465822,-2.1));
#64665=CARTESIAN_POINT('',(29.6403124237433,-7.8,-2.));
#64666=CARTESIAN_POINT('Origin',(29.,-7.8,0.));
#64667=CARTESIAN_POINT('',(29.6403124237433,-6.72842712474619,-2.));
#64668=CARTESIAN_POINT('',(28.3596875762567,-7.8,-2.));
#64669=CARTESIAN_POINT('',(28.3596875762567,-6.72842712474619,-2.));
#64670=CARTESIAN_POINT('',(28.3596875762567,-7.8,2.));
#64671=CARTESIAN_POINT('Origin',(29.,-7.8,0.));
#64672=CARTESIAN_POINT('',(28.3596875762567,-6.72842712474619,2.));
#64673=CARTESIAN_POINT('',(29.6403124237433,-6.72842712474619,2.));
#64674=CARTESIAN_POINT('Origin',(24.,-3.9,-2.));
#64675=CARTESIAN_POINT('',(24.,-7.8,-2.));
#64676=CARTESIAN_POINT('Origin',(24.,-3.9,-2.));
#64677=CARTESIAN_POINT('',(24.,-7.8,-2.));
#64678=CARTESIAN_POINT('Origin',(24.,-7.8,0.));
#64679=CARTESIAN_POINT('',(24.,-7.8,2.));
#64680=CARTESIAN_POINT('Origin',(24.,-7.8,0.));
#64681=CARTESIAN_POINT('',(24.,-7.8,2.));
#64682=CARTESIAN_POINT('Origin',(24.,-3.9,2.));
#64683=CARTESIAN_POINT('Origin',(24.,-3.9,2.));
#64684=CARTESIAN_POINT('Origin',(1.,0.,22.5));
#64685=CARTESIAN_POINT('',(-7.,-12.8747815515449,24.3));
#64686=CARTESIAN_POINT('',(-7.,-10.0876161703348,14.3));
#64687=CARTESIAN_POINT('Origin',(-7.,0.,22.5));
#64688=CARTESIAN_POINT('',(1.,-12.8747815515449,24.3));
#64689=CARTESIAN_POINT('',(1.,-10.0876161703348,14.3));
#64690=CARTESIAN_POINT('Origin',(1.,-22.5,0.));
#64691=CARTESIAN_POINT('',(-7.,-24.3,-12.8747815515449));
#64692=CARTESIAN_POINT('',(-7.,-14.3,-10.0876161703348));
#64693=CARTESIAN_POINT('Origin',(-7.,-22.5,0.));
#64694=CARTESIAN_POINT('',(1.,-24.3,-12.8747815515449));
#64695=CARTESIAN_POINT('',(1.,-14.3,-10.0876161703348));
#64696=CARTESIAN_POINT('Origin',(1.,0.,-22.5));
#64697=CARTESIAN_POINT('',(-7.,-12.8747815515449,-24.3));
#64698=CARTESIAN_POINT('',(1.,-12.8747815515449,-24.3));
#64699=CARTESIAN_POINT('',(-7.,-10.0876161703348,-14.3));
#64700=CARTESIAN_POINT('Origin',(-7.,0.,-22.5));
#64701=CARTESIAN_POINT('',(1.,-10.0876161703348,-14.3));
#64702=CARTESIAN_POINT('Origin',(1.,0.,0.));
#64703=CARTESIAN_POINT('',(-7.,-14.3,10.0876161703348));
#64704=CARTESIAN_POINT('Origin',(-7.,0.,0.));
#64705=CARTESIAN_POINT('',(1.,-14.3,10.0876161703348));
#64706=CARTESIAN_POINT('Origin',(1.,0.,0.));
#64707=CARTESIAN_POINT('Origin',(-7.,0.,0.));
#64708=CARTESIAN_POINT('Origin',(1.,-22.5,0.));
#64709=CARTESIAN_POINT('',(-7.,-24.3,12.8747815515449));
#64710=CARTESIAN_POINT('',(1.,-24.3,12.8747815515449));
#64711=CARTESIAN_POINT('Origin',(-7.,-22.5,0.));
#64712=CARTESIAN_POINT('Origin',(-7.,-9.72271824131503,9.72271824131503));
#64713=CARTESIAN_POINT('Origin',(-7.,0.,0.));
#64714=CARTESIAN_POINT('Origin',(-7.,-9.72271824131503,9.72271824131503));
#64715=CARTESIAN_POINT('Origin',(-7.,0.,0.));
#64716=CARTESIAN_POINT('Origin',(15.25,0.,0.));
#64717=CARTESIAN_POINT('',(4.3435534146,-17.874107980537,20.8989536556285));
#64718=CARTESIAN_POINT('',(5.18767834635794,-19.7673317665207,19.118122157584));
#64719=CARTESIAN_POINT('Ctrl Pts',(5.18767834635793,-19.7673317665207,19.118122157584));
#64720=CARTESIAN_POINT('Ctrl Pts',(5.24965809277247,-19.7360217070282,19.1504954382083));
#64721=CARTESIAN_POINT('Ctrl Pts',(5.30712124170086,-19.7015935906934,19.1859300894978));
#64722=CARTESIAN_POINT('Ctrl Pts',(5.48660165044913,-19.5761078943939,19.3143019932782));
#64723=CARTESIAN_POINT('Ctrl Pts',(5.59711475871681,-19.4625384572688,19.4291249072538));
#64724=CARTESIAN_POINT('Ctrl Pts',(5.74364605565176,-19.2109564252457,19.6779178545318));
#64725=CARTESIAN_POINT('Ctrl Pts',(5.7796645257,-19.0728726925368,19.8118157765002));
#64726=CARTESIAN_POINT('Ctrl Pts',(5.7796645257,-18.8112850369902,20.060362407785));
#64727=CARTESIAN_POINT('Ctrl Pts',(5.74357914128895,-18.6703688818376,20.1915501172113));
#64728=CARTESIAN_POINT('Ctrl Pts',(5.59693543031386,-18.408739121605,20.4303620690589));
#64729=CARTESIAN_POINT('Ctrl Pts',(5.4863803371174,-18.2880926642702,20.5380618497645));
#64730=CARTESIAN_POINT('Ctrl Pts',(5.2314028462211,-18.0965825390734,20.7070034351683));
#64731=CARTESIAN_POINT('Ctrl Pts',(5.06999631183931,-18.0129189000428,20.779560855588));
#64732=CARTESIAN_POINT('Ctrl Pts',(4.71625542419336,-17.90164394286,20.8755009713159));
#64733=CARTESIAN_POINT('Ctrl Pts',(4.52391635613999,-17.874107980537,20.8989536556285));
#64734=CARTESIAN_POINT('Ctrl Pts',(4.3435534146,-17.874107980537,20.8989536556285));
#64735=CARTESIAN_POINT('',(5.7631397208,-20.8989536556285,17.874107980537));
#64736=CARTESIAN_POINT('Origin',(5.03051074633478,2.27365790259165,-2.27404388388516));
#64737=CARTESIAN_POINT('',(4.7295794663,-20.8989536556285,17.874107980537));
#64738=CARTESIAN_POINT('',(5.24635959355,-20.8989536556285,17.874107980537));
#64739=CARTESIAN_POINT('',(4.2292347159,-19.9191739484904,18.9598657487278));
#64740=CARTESIAN_POINT('Origin',(3.9969811813217,2.27238339981618,-2.27289593102036));
#64741=CARTESIAN_POINT('',(3.7202200813,-19.9191739484904,18.9598657487278));
#64742=CARTESIAN_POINT('',(3.9747273986,-19.9191739484904,18.9598657487278));
#64743=CARTESIAN_POINT('',(3.7202200813,-20.8989536556285,17.874107980537));
#64744=CARTESIAN_POINT('Origin',(3.7202200813,0.,0.));
#64745=CARTESIAN_POINT('',(2.7424423035,-20.8989536556285,17.874107980537));
#64746=CARTESIAN_POINT('',(3.2313311924,-20.8989536556285,17.874107980537));
#64747=CARTESIAN_POINT('',(2.7424423035,-17.874107980537,20.8989536556285));
#64748=CARTESIAN_POINT('Origin',(2.7424423035,0.,0.));
#64749=CARTESIAN_POINT('',(3.54299785905,-17.874107980537,20.8989536556285));
#64750=CARTESIAN_POINT('',(1.4888888889,-18.6070663646292,20.2491254453689));
#64751=CARTESIAN_POINT('',(1.4888888889,-20.8989536556285,17.874107980537));
#64752=CARTESIAN_POINT('Origin',(1.4888888889,0.,0.));
#64753=CARTESIAN_POINT('',(0.5111111111,-20.8989536556285,17.874107980537));
#64754=CARTESIAN_POINT('',(1.,-20.8989536556285,17.874107980537));
#64755=CARTESIAN_POINT('',(0.5111111111,-18.6070663646292,20.2491254453689));
#64756=CARTESIAN_POINT('Origin',(0.5111111111,0.,0.));
#64757=CARTESIAN_POINT('',(-0.5277777778,-18.6070663646292,20.2491254453689));
#64758=CARTESIAN_POINT('',(-0.00833333335000042,-18.6070663646292,20.2491254453689));
#64759=CARTESIAN_POINT('',(-0.5277777778,-17.874107980537,20.8989536556285));
#64760=CARTESIAN_POINT('Origin',(-0.527777777800001,0.,0.));
#64761=CARTESIAN_POINT('',(2.5277777778,-17.874107980537,20.8989536556285));
#64762=CARTESIAN_POINT('',(1.,-17.874107980537,20.8989536556285));
#64763=CARTESIAN_POINT('',(2.5277777778,-18.6070663646292,20.2491254453689));
#64764=CARTESIAN_POINT('Origin',(2.5277777778,0.,0.));
#64765=CARTESIAN_POINT('',(2.00833333335,-18.6070663646292,20.2491254453689));
#64766=CARTESIAN_POINT('',(-3.7631397208,-21.2925086575347,17.4034213610087));
#64767=CARTESIAN_POINT('',(-1.8075841652,-21.2925086575347,17.4034213610087));
#64768=CARTESIAN_POINT('',(-2.785361943,-21.2925086575347,17.4034213610086));
#64769=CARTESIAN_POINT('',(1.,-22.2889734574269,16.1075032892786));
#64770=CARTESIAN_POINT('Origin',(-6.57072387330978,-4.43551506634776E-8,
3.4092084710835E-8));
#64771=CARTESIAN_POINT('',(3.8075841652,-21.2925086575347,17.4034213610087));
#64772=CARTESIAN_POINT('Origin',(8.57072389460998,2.73287437124736E-8,-2.01895722362622E-8));
#64773=CARTESIAN_POINT('',(5.7631397208,-21.2925086575347,17.4034213610087));
#64774=CARTESIAN_POINT('',(4.785361943,-21.2925086575347,17.4034213610086));
#64775=CARTESIAN_POINT('',(1.,-22.9416461797837,15.1634715867317));
#64776=CARTESIAN_POINT('Origin',(10.5262794394392,-7.77399478124607E-9,
6.01586114257202E-9));
#64777=CARTESIAN_POINT('Origin',(-8.52627944622453,1.44232226162444E-8,
-1.06424180579268E-8));
#64778=CARTESIAN_POINT('',(-1.9747474276,-19.3023137418562,19.5875134769819));
#64779=CARTESIAN_POINT('',(-0.5561396937,-20.8989536556285,17.874107980537));
#64780=CARTESIAN_POINT('Origin',(-1.85251751839491,0.,0.));
#64781=CARTESIAN_POINT('',(-1.6994942043,-20.8989536556285,17.874107980537));
#64782=CARTESIAN_POINT('',(-1.127816949,-20.8989536556285,17.874107980537));
#64783=CARTESIAN_POINT('',(-2.785361943,-19.6894777136292,19.1982933450997));
#64784=CARTESIAN_POINT('Origin',(-2.99551159274116,7.11916623071864,-7.12000723870792));
#64785=CARTESIAN_POINT('',(-2.785361943,-20.8989536556285,17.874107980537));
#64786=CARTESIAN_POINT('Origin',(-2.785361943,0.,0.));
#64787=CARTESIAN_POINT('',(-3.7631397208,-20.8989536556285,17.874107980537));
#64788=CARTESIAN_POINT('',(-3.2742508319,-20.8989536556285,17.874107980537));
#64789=CARTESIAN_POINT('',(-3.7631397208,-17.874107980537,20.8989536556285));
#64790=CARTESIAN_POINT('Origin',(-3.7631397208,0.,0.));
#64791=CARTESIAN_POINT('',(-2.785361943,-17.874107980537,20.8989536556285));
#64792=CARTESIAN_POINT('',(-3.2742508319,-17.874107980537,20.8989536556285));
#64793=CARTESIAN_POINT('',(-2.785361943,-18.9090114682761,19.9674556539536));
#64794=CARTESIAN_POINT('Origin',(-2.785361943,0.,0.));
#64795=CARTESIAN_POINT('',(-1.8474876449,-17.874107980537,20.8989536556285));
#64796=CARTESIAN_POINT('Origin',(-3.28939526749656,8.80977299836507,-8.80811422836384));
#64797=CARTESIAN_POINT('',(-0.6680745397,-17.874107980537,20.8989536556285));
#64798=CARTESIAN_POINT('',(-1.2577810923,-17.874107980537,20.8989536556285));
#64799=CARTESIAN_POINT('Origin',(-2.11077331185338,0.,0.));
#64800=CARTESIAN_POINT('',(1.,-16.1075032892786,22.2889734574269));
#64801=CARTESIAN_POINT('',(-1.8075841652,-17.4034213610087,21.2925086575347));
#64802=CARTESIAN_POINT('Origin',(-6.5707239016573,3.78664832823006E-8,-5.07550401707135E-8));
#64803=CARTESIAN_POINT('',(-3.7631397208,-17.4034213610087,21.2925086575347));
#64804=CARTESIAN_POINT('',(-2.785361943,-17.4034213610086,21.2925086575347));
#64805=CARTESIAN_POINT('',(1.,-15.1634715867317,22.9416461797837));
#64806=CARTESIAN_POINT('Origin',(-8.52627943980808,-4.20687484847804E-9,
5.66308777649738E-9));
#64807=CARTESIAN_POINT('',(5.7631397208,-17.4034213610087,21.2925086575347));
#64808=CARTESIAN_POINT('Origin',(10.5262794297275,-2.73344635814965E-8,
3.70220565315549E-8));
#64809=CARTESIAN_POINT('',(3.8075841652,-17.4034213610087,21.2925086575347));
#64810=CARTESIAN_POINT('',(4.785361943,-17.4034213610086,21.2925086575347));
#64811=CARTESIAN_POINT('Origin',(8.57072386182903,-7.01216418264039E-8,
8.97514196296356E-8));
#64812=CARTESIAN_POINT('Origin',(1.,0.,0.));
#64813=CARTESIAN_POINT('',(1.4888888889,-20.5443060118528,17.5194603367613));
#64814=CARTESIAN_POINT('',(1.4888888889,-18.2531915575896,19.8952506383293));
#64815=CARTESIAN_POINT('Origin',(1.4888888889,0.,0.));
#64816=CARTESIAN_POINT('',(2.5277777778,-18.2531915575896,19.8952506383293));
#64817=CARTESIAN_POINT('',(2.00833333335,-18.2531915575896,19.8952506383293));
#64818=CARTESIAN_POINT('',(2.5277777778,-17.5194603367613,20.5443060118528));
#64819=CARTESIAN_POINT('Origin',(2.5277777778,0.,0.));
#64820=CARTESIAN_POINT('',(-0.5277777778,-17.5194603367613,20.5443060118528));
#64821=CARTESIAN_POINT('',(1.,-17.5194603367613,20.5443060118528));
#64822=CARTESIAN_POINT('',(-0.5277777778,-18.2531915575896,19.8952506383293));
#64823=CARTESIAN_POINT('Origin',(-0.527777777800001,0.,0.));
#64824=CARTESIAN_POINT('',(0.5111111111,-18.2531915575896,19.8952506383293));
#64825=CARTESIAN_POINT('',(-0.00833333335000086,-18.2531915575896,19.8952506383293));
#64826=CARTESIAN_POINT('',(0.5111111111,-20.5443060118528,17.5194603367613));
#64827=CARTESIAN_POINT('Origin',(0.5111111111,0.,0.));
#64828=CARTESIAN_POINT('',(1.,-20.5443060118528,17.5194603367613));
#64829=CARTESIAN_POINT('Origin',(0.5111111111,-0.345696648587947,-0.345696648587947));
#64830=CARTESIAN_POINT('',(0.5111111111,-1.51242283754575,-1.51242283754575));
#64831=CARTESIAN_POINT('',(0.5111111111,0.821029540369857,0.821029540369857));
#64832=CARTESIAN_POINT('Origin',(1.,-1.51242283754575,-1.51242283754575));
#64833=CARTESIAN_POINT('',(1.4888888889,-1.51242283754575,-1.51242283754575));
#64834=CARTESIAN_POINT('Origin',(-0.00833333334999997,0.821029540369857,
0.821029540369857));
#64835=CARTESIAN_POINT('',(-0.5277777778,0.821029540369857,0.821029540369857));
#64836=CARTESIAN_POINT('Origin',(-0.5277777778,1.1667261889578,1.1667261889578));
#64837=CARTESIAN_POINT('',(-0.5277777778,1.51242283754575,1.51242283754575));
#64838=CARTESIAN_POINT('Origin',(1.,1.51242283754575,1.51242283754575));
#64839=CARTESIAN_POINT('',(2.5277777778,1.51242283754575,1.51242283754575));
#64840=CARTESIAN_POINT('Origin',(2.5277777778,1.1667261889578,1.1667261889578));
#64841=CARTESIAN_POINT('',(2.5277777778,0.821029540369857,0.821029540369857));
#64842=CARTESIAN_POINT('Origin',(2.00833333335,0.821029540369857,0.821029540369857));
#64843=CARTESIAN_POINT('',(1.4888888889,0.821029540369857,0.821029540369857));
#64844=CARTESIAN_POINT('Origin',(1.4888888889,-0.345696648587947,-0.345696648587947));
#64845=CARTESIAN_POINT('Origin',(-2.24242807365,-0.879007510905235,-0.879007510905235));
#64846=CARTESIAN_POINT('',(-1.6994942043,-20.5443060118528,17.5194603367613));
#64847=CARTESIAN_POINT('',(-1.6994942043,-1.51242283754575,-1.51242283754575));
#64848=CARTESIAN_POINT('',(-2.785361943,-19.3358955993241,18.8447112307947));
#64849=CARTESIAN_POINT('Origin',(-2.99587202900024,0.,0.));
#64850=CARTESIAN_POINT('',(-2.785361943,-0.245592184264721,-0.245592184264721));
#64851=CARTESIAN_POINT('Origin',(-1.127816949,-1.51242283754575,-1.51242283754575));
#64852=CARTESIAN_POINT('',(-0.5561396937,-20.5443060118528,17.5194603367613));
#64853=CARTESIAN_POINT('',(-0.5561396937,-1.51242283754575,-1.51242283754575));
#64854=CARTESIAN_POINT('',(-1.127816949,-20.5443060118528,17.5194603367613));
#64855=CARTESIAN_POINT('Origin',(-1.26544356065,-0.684911484991446,-0.684911484991446));
#64856=CARTESIAN_POINT('',(-1.9747474276,-18.9487506681581,19.2339504032838));
#64857=CARTESIAN_POINT('',(-1.9747474276,0.142599867562857,0.142599867562857));
#64858=CARTESIAN_POINT('Origin',(-1.85251751839491,0.,0.));
#64859=CARTESIAN_POINT('Origin',(-1.2577810923,1.51242283754575,1.51242283754575));
#64860=CARTESIAN_POINT('',(-1.8474876449,-17.5194603367613,20.5443060118528));
#64861=CARTESIAN_POINT('',(-1.8474876449,1.51242283754575,1.51242283754575));
#64862=CARTESIAN_POINT('',(-0.6680745397,-17.5194603367613,20.5443060118528));
#64863=CARTESIAN_POINT('',(-1.2577810923,-17.5194603367613,20.5443060118528));
#64864=CARTESIAN_POINT('',(-0.6680745397,1.51242283754575,1.51242283754575));
#64865=CARTESIAN_POINT('Origin',(-2.31642479395,1.02082246519224,1.02082246519224));
#64866=CARTESIAN_POINT('',(-2.785361943,-18.5553246394379,19.6137688251154));
#64867=CARTESIAN_POINT('',(-2.785361943,0.529222092838726,0.529222092838726));
#64868=CARTESIAN_POINT('Origin',(-3.28936566907665,8.64824730080475,-8.6465264730355));
#64869=CARTESIAN_POINT('Origin',(-2.785361943,1.02082246519224,1.02082246519224));
#64870=CARTESIAN_POINT('',(-2.785361943,-17.5194603367613,20.5443060118528));
#64871=CARTESIAN_POINT('',(-2.785361943,1.51242283754575,1.51242283754575));
#64872=CARTESIAN_POINT('Origin',(-2.785361943,0.,0.));
#64873=CARTESIAN_POINT('Origin',(-3.2742508319,1.51242283754575,1.51242283754575));
#64874=CARTESIAN_POINT('',(-3.7631397208,-17.5194603367613,20.5443060118528));
#64875=CARTESIAN_POINT('',(-3.7631397208,1.51242283754575,1.51242283754575));
#64876=CARTESIAN_POINT('',(-3.2742508319,-17.5194603367613,20.5443060118528));
#64877=CARTESIAN_POINT('Origin',(-3.7631397208,0.,0.));
#64878=CARTESIAN_POINT('',(-3.7631397208,-20.5443060118528,17.5194603367613));
#64879=CARTESIAN_POINT('',(-3.7631397208,-1.51242283754575,-1.51242283754575));
#64880=CARTESIAN_POINT('Origin',(-3.7631397208,0.,0.));
#64881=CARTESIAN_POINT('Origin',(-3.2742508319,-1.51242283754575,-1.51242283754575));
#64882=CARTESIAN_POINT('',(-2.785361943,-20.5443060118528,17.5194603367613));
#64883=CARTESIAN_POINT('',(-2.785361943,-1.51242283754575,-1.51242283754575));
#64884=CARTESIAN_POINT('',(-3.2742508319,-20.5443060118528,17.5194603367613));
#64885=CARTESIAN_POINT('Origin',(-2.785361943,-0.879007510905235,-0.879007510905235));
#64886=CARTESIAN_POINT('Origin',(-2.785361943,0.,0.));
#64887=CARTESIAN_POINT('Origin',(-1.32141098365,0.827511352554304,0.827511352554304));
#64888=CARTESIAN_POINT('Origin',(-2.11077331185338,0.,0.));
#64889=CARTESIAN_POINT('Origin',(1.,0.,0.));
#64890=CARTESIAN_POINT('Origin',(1.,0.,0.));
#64891=CARTESIAN_POINT('',(1.,-22.5806629390448,14.8024883459927));
#64892=CARTESIAN_POINT('',(5.7631397208,-20.9371408903466,17.0480535938206));
#64893=CARTESIAN_POINT('Origin',(10.526279445577,1.21171739309034E-8,-8.89615270338595E-9));
#64894=CARTESIAN_POINT('',(3.8075841652,-20.9371408903466,17.0480535938206));
#64895=CARTESIAN_POINT('',(4.785361943,-20.9371408903466,17.0480535938206));
#64896=CARTESIAN_POINT('',(1.,-21.930781703976,15.7493115358277));
#64897=CARTESIAN_POINT('Origin',(8.57072385391719,-1.12072822133769E-7,
8.59802584685099E-8));
#64898=CARTESIAN_POINT('',(-1.8075841652,-20.9371408903466,17.0480535938206));
#64899=CARTESIAN_POINT('Origin',(-6.57072381790309,-2.36861166236224E-7,
1.81346071492783E-7));
#64900=CARTESIAN_POINT('',(-3.7631397208,-20.9371408903466,17.0480535938206));
#64901=CARTESIAN_POINT('',(-2.785361943,-20.9371408903466,17.0480535938206));
#64902=CARTESIAN_POINT('Origin',(-8.52627944430539,8.13953349165786E-9,
-5.95527405167218E-9));
#64903=CARTESIAN_POINT('Origin',(2.4037920826,-2.51763936616857,-2.51763936616857));
#64904=CARTESIAN_POINT('',(1.,-3.09073508407414,-3.09073508407414));
#64905=CARTESIAN_POINT('',(3.8075841652,-1.94454364826301,-1.94454364826301));
#64906=CARTESIAN_POINT('Origin',(-0.4037920826,-2.51763936616857,-2.51763936616857));
#64907=CARTESIAN_POINT('',(-1.8075841652,-1.94454364826301,-1.94454364826301));
#64908=CARTESIAN_POINT('Origin',(4.785361943,-1.94454364826301,-1.94454364826301));
#64909=CARTESIAN_POINT('',(5.7631397208,-1.94454364826301,-1.94454364826301));
#64910=CARTESIAN_POINT('Origin',(3.3815698604,-2.91681547239451,-2.91681547239451));
#64911=CARTESIAN_POINT('',(1.,-3.88908729652601,-3.88908729652601));
#64912=CARTESIAN_POINT('Origin',(-1.3815698604,-2.91681547239451,-2.91681547239451));
#64913=CARTESIAN_POINT('',(-3.7631397208,-1.94454364826301,-1.94454364826301));
#64914=CARTESIAN_POINT('Origin',(-2.785361943,-1.94454364826301,-1.94454364826301));
#64915=CARTESIAN_POINT('Origin',(4.785361943,1.94454364826301,1.94454364826301));
#64916=CARTESIAN_POINT('',(5.7631397208,-17.0480535938206,20.9371408903466));
#64917=CARTESIAN_POINT('',(5.7631397208,1.94454364826301,1.94454364826301));
#64918=CARTESIAN_POINT('',(3.8075841652,-17.0480535938206,20.9371408903466));
#64919=CARTESIAN_POINT('',(4.785361943,-17.0480535938206,20.9371408903466));
#64920=CARTESIAN_POINT('',(3.8075841652,1.94454364826301,1.94454364826301));
#64921=CARTESIAN_POINT('Origin',(3.3815698604,2.91681547239451,2.91681547239451));
#64922=CARTESIAN_POINT('',(1.,-14.8024883459927,22.5806629390448));
#64923=CARTESIAN_POINT('',(1.,3.88908729652601,3.88908729652601));
#64924=CARTESIAN_POINT('Origin',(10.5262794421488,1.26208155037943E-9,-1.68191238714144E-9));
#64925=CARTESIAN_POINT('Origin',(-1.3815698604,2.91681547239451,2.91681547239451));
#64926=CARTESIAN_POINT('',(-3.7631397208,-17.0480535938206,20.9371408903466));
#64927=CARTESIAN_POINT('',(-3.7631397208,1.94454364826301,1.94454364826301));
#64928=CARTESIAN_POINT('Origin',(-8.52627944021436,-3.35364402914706E-9,
4.51061854533918E-9));
#64929=CARTESIAN_POINT('Origin',(-2.785361943,1.94454364826301,1.94454364826301));
#64930=CARTESIAN_POINT('',(-1.8075841652,-17.0480535938206,20.9371408903466));
#64931=CARTESIAN_POINT('',(-1.8075841652,1.94454364826301,1.94454364826301));
#64932=CARTESIAN_POINT('',(-2.785361943,-17.0480535938206,20.9371408903466));
#64933=CARTESIAN_POINT('Origin',(2.4037920826,2.51763936616857,2.51763936616857));
#64934=CARTESIAN_POINT('',(1.,-15.7493115358277,21.930781703976));
#64935=CARTESIAN_POINT('Origin',(8.57072390411113,4.73520644916903E-8,-6.22505558212083E-8));
#64936=CARTESIAN_POINT('',(1.,3.09073508407414,3.09073508407414));
#64937=CARTESIAN_POINT('Origin',(-0.4037920826,2.51763936616857,2.51763936616857));
#64938=CARTESIAN_POINT('Origin',(-6.57072389687678,3.12376124966818E-8,
-4.02133704113794E-8));
#64939=CARTESIAN_POINT('Origin',(1.,0.,0.));
#64940=CARTESIAN_POINT('Origin',(4.4794070911,-0.996038468713527,-0.996038468713527));
#64941=CARTESIAN_POINT('',(4.7295794663,-20.5443060118528,17.5194603367613));
#64942=CARTESIAN_POINT('',(4.7295794663,-1.51242283754575,-1.51242283754575));
#64943=CARTESIAN_POINT('',(4.2292347159,-19.56551095632,18.6062027565574));
#64944=CARTESIAN_POINT('Origin',(3.99698582654048,2.23070863740945,-2.23124034514977));
#64945=CARTESIAN_POINT('',(4.2292347159,-0.479654099881305,-0.479654099881305));
#64946=CARTESIAN_POINT('Origin',(5.24635959355,-1.51242283754575,-1.51242283754575));
#64947=CARTESIAN_POINT('',(5.7631397208,-20.5443060118528,17.5194603367613));
#64948=CARTESIAN_POINT('',(5.7631397208,-1.51242283754575,-1.51242283754575));
#64949=CARTESIAN_POINT('',(5.24635959355,-20.5443060118528,17.5194603367613));
#64950=CARTESIAN_POINT('Origin',(5.47540903359635,-0.918513821002833,-0.918513821002833));
#64951=CARTESIAN_POINT('',(5.18767834635794,-19.4137281924324,18.7645185834957));
#64952=CARTESIAN_POINT('',(5.18767834635794,-0.324604804468337,-0.324604804468337));
#64953=CARTESIAN_POINT('Origin',(5.03051424672319,2.23200783897291,-2.23240826550412));
#64954=CARTESIAN_POINT('Origin',(4.3435534146,0.496938932349593,0.496938932349593));
#64955=CARTESIAN_POINT('',(4.3435534146,-17.5194603367613,20.5443060118528));
#64956=CARTESIAN_POINT('',(4.3435534146,1.51242283754575,1.51242283754575));
#64957=CARTESIAN_POINT('Ctrl Pts',(4.3435534146,-17.5194603367613,20.5443060118528));
#64958=CARTESIAN_POINT('Ctrl Pts',(4.52391792341369,-17.5194603367613,20.5443060118528));
#64959=CARTESIAN_POINT('Ctrl Pts',(4.71625693450842,-17.5470348446854,20.5208909607321));
#64960=CARTESIAN_POINT('Ctrl Pts',(5.06999455179236,-17.6584515309732,20.4250945452161));
#64961=CARTESIAN_POINT('Ctrl Pts',(5.23139805095757,-17.7422168695679,20.3526419083133));
#64962=CARTESIAN_POINT('Ctrl Pts',(5.48637421277749,-17.9339330499853,20.1839135315558));
#64963=CARTESIAN_POINT('Ctrl Pts',(5.59693050287028,-18.0546991682471,20.0763345995508));
#64964=CARTESIAN_POINT('Ctrl Pts',(5.74357733669248,-18.3165417747782,19.8377335001105));
#64965=CARTESIAN_POINT('Ctrl Pts',(5.7796645257,-18.4575499635599,19.7066343295773));
#64966=CARTESIAN_POINT('Ctrl Pts',(5.7796645257,-18.71926054171,19.4582065445153));
#64967=CARTESIAN_POINT('Ctrl Pts',(5.7436467578758,-18.8573825010707,19.3243479332158));
#64968=CARTESIAN_POINT('Ctrl Pts',(5.59711654864042,-19.1089901329801,19.0755810903176));
#64969=CARTESIAN_POINT('Ctrl Pts',(5.48660381528006,-19.2225482493687,18.9607463124921));
#64970=CARTESIAN_POINT('Ctrl Pts',(5.30712307306233,-19.3480080907561,18.8323468119573));
#64971=CARTESIAN_POINT('Ctrl Pts',(5.24965906631464,-19.3824274887551,18.7969022202364));
#64972=CARTESIAN_POINT('Ctrl Pts',(5.18767834635793,-19.4137281924324,18.7645185834957));
#64973=CARTESIAN_POINT('Origin',(3.54299785905,1.51242283754575,1.51242283754575));
#64974=CARTESIAN_POINT('',(2.7424423035,-17.5194603367613,20.5443060118528));
#64975=CARTESIAN_POINT('',(2.7424423035,1.51242283754575,1.51242283754575));
#64976=CARTESIAN_POINT('',(3.54299785905,-17.5194603367613,20.5443060118528));
#64977=CARTESIAN_POINT('Origin',(3.7202200813,0.496938932349593,0.496938932349593));
#64978=CARTESIAN_POINT('',(3.7202200813,-18.2937167290108,19.85799406382));
#64979=CARTESIAN_POINT('',(3.7202200813,0.782138667404597,0.782138667404597));
#64980=CARTESIAN_POINT('',(3.7202200813,-18.8789697081476,19.3024481027368));
#64981=CARTESIAN_POINT('Origin',(3.7202200813,0.,0.));
#64982=CARTESIAN_POINT('',(3.7202200813,0.211739197294589,0.211739197294589));
#64983=CARTESIAN_POINT('Origin',(4.03188674795,0.782138667404597,0.782138667404597));
#64984=CARTESIAN_POINT('',(4.3435534146,-18.2937167290108,19.85799406382));
#64985=CARTESIAN_POINT('',(4.3435534146,0.782138667404597,0.782138667404597));
#64986=CARTESIAN_POINT('',(4.03188674795,-18.2937167290108,19.85799406382));
#64987=CARTESIAN_POINT('Origin',(2.7424423035,0.,0.));
#64988=CARTESIAN_POINT('',(2.7424423035,-20.5443060118528,17.5194603367613));
#64989=CARTESIAN_POINT('',(2.7424423035,-1.51242283754575,-1.51242283754575));
#64990=CARTESIAN_POINT('Origin',(2.7424423035,0.,0.));
#64991=CARTESIAN_POINT('Origin',(3.2313311924,-1.51242283754575,-1.51242283754575));
#64992=CARTESIAN_POINT('',(3.7202200813,-20.5443060118528,17.5194603367613));
#64993=CARTESIAN_POINT('',(3.7202200813,-1.51242283754575,-1.51242283754575));
#64994=CARTESIAN_POINT('',(3.2313311924,-20.5443060118528,17.5194603367613));
#64995=CARTESIAN_POINT('Origin',(3.7202200813,-0.996038468713527,-0.996038468713527));
#64996=CARTESIAN_POINT('',(3.7202200813,-19.56551095632,18.6062027565574));
#64997=CARTESIAN_POINT('',(3.7202200813,-0.479654099881305,-0.479654099881305));
#64998=CARTESIAN_POINT('Origin',(3.7202200813,0.,0.));
#64999=CARTESIAN_POINT('Origin',(3.9747273986,-0.479654099881305,-0.479654099881305));
#65000=CARTESIAN_POINT('',(3.9747273986,-19.56551095632,18.6062027565574));
#65001=CARTESIAN_POINT('Origin',(4.3435534146,0.496938932349593,0.496938932349593));
#65002=CARTESIAN_POINT('',(4.3435534146,-18.8789697081476,19.3024481027368));
#65003=CARTESIAN_POINT('',(4.3435534146,0.211739197294589,0.211739197294589));
#65004=CARTESIAN_POINT('Ctrl Pts',(4.3435534146,-18.2937167290108,19.85799406382));
#65005=CARTESIAN_POINT('Ctrl Pts',(4.39419751981262,-18.2937167290108,19.85799406382));
#65006=CARTESIAN_POINT('Ctrl Pts',(4.44821399727505,-18.3011713769004,19.8511347365578));
#65007=CARTESIAN_POINT('Ctrl Pts',(4.54757547767286,-18.3314319885872,19.8231941256532));
#65008=CARTESIAN_POINT('Ctrl Pts',(4.59292073016298,-18.3542319727212,19.8021072538948));
#65009=CARTESIAN_POINT('Ctrl Pts',(4.66454409879151,-18.40672084645,19.7533266057787));
#65010=CARTESIAN_POINT('Ctrl Pts',(4.69559097470685,-18.4399132778847,19.7223748562545));
#65011=CARTESIAN_POINT('Ctrl Pts',(4.73676234178596,-18.5124187162062,19.6543334901588));
#65012=CARTESIAN_POINT('Ctrl Pts',(4.7468867479,-18.5517261768333,19.617237912228));
#65013=CARTESIAN_POINT('Ctrl Pts',(4.7468867479,-18.625214121851,19.5474797559526));
#65014=CARTESIAN_POINT('Ctrl Pts',(4.73676781048986,-18.6642939918242,19.5101665751395));
#65015=CARTESIAN_POINT('Ctrl Pts',(4.69560563233662,-18.7359923229461,19.441323557758));
#65016=CARTESIAN_POINT('Ctrl Pts',(4.66456218935101,-18.7686163667244,19.4097996565274));
#65017=CARTESIAN_POINT('Ctrl Pts',(4.59293647859085,-18.8200438549336,19.3599388355082));
#65018=CARTESIAN_POINT('Ctrl Pts',(4.54758424200201,-18.8422779900643,19.3382776827266));
#65019=CARTESIAN_POINT('Ctrl Pts',(4.44821398195441,-18.8717380395622,19.3095294338108));
#65020=CARTESIAN_POINT('Ctrl Pts',(4.39419599674402,-18.8789697081476,19.3024481027368));
#65021=CARTESIAN_POINT('Ctrl Pts',(4.3435534146,-18.8789697081476,19.3024481027368));
#65022=CARTESIAN_POINT('Origin',(4.03188674795,0.211739197294589,0.211739197294589));
#65023=CARTESIAN_POINT('',(4.03188674795,-18.8789697081476,19.3024481027368));
#65024=CARTESIAN_POINT('Origin',(1.,0.,0.));
#66670=UNCERTAINTY_MEASURE_WITH_UNIT(LENGTH_MEASURE(0.01),#66722,
'DISTANCE_ACCURACY_VALUE',
'Maximum model space distance between geometric entities at asserted c
onnectivities');
#66680=UNCERTAINTY_MEASURE_WITH_UNIT(LENGTH_MEASURE(0.01),#66722,
'DISTANCE_ACCURACY_VALUE',
'Maximum model space distance between geometric entities at asserted c
onnectivities');
#66711=(
GEOMETRIC_REPRESENTATION_CONTEXT(3)
GLOBAL_UNCERTAINTY_ASSIGNED_CONTEXT((#66670))
GLOBAL_UNIT_ASSIGNED_CONTEXT((#66722,#66724,#66725))
REPRESENTATION_CONTEXT('','3D')
);
#66721=(
GEOMETRIC_REPRESENTATION_CONTEXT(3)
GLOBAL_UNCERTAINTY_ASSIGNED_CONTEXT((#66680))
GLOBAL_UNIT_ASSIGNED_CONTEXT((#66722,#66724,#66725))
REPRESENTATION_CONTEXT('','3D')
);
#66722=(
LENGTH_UNIT()
NAMED_UNIT(*)
SI_UNIT(.MILLI.,.METRE.)
);
#66724=(
NAMED_UNIT(*)
PLANE_ANGLE_UNIT()
SI_UNIT($,.RADIAN.)
);
#66725=(
NAMED_UNIT(*)
SI_UNIT($,.STERADIAN.)
SOLID_ANGLE_UNIT()
);
#66756=SHAPE_DEFINITION_REPRESENTATION(#66816,#66920);
#66816=PRODUCT_DEFINITION_SHAPE('',$,#66961);
#66920=SHAPE_REPRESENTATION('',(#28001),#66711);
#66930=PRODUCT_DEFINITION_CONTEXT('part definition',#67052,'design');
#66961=PRODUCT_DEFINITION('Coupling Hub 2','Coupling Hub 2',#67001,#66930);
#67001=PRODUCT_DEFINITION_FORMATION('',$,#67084);
#67052=APPLICATION_CONTEXT(
'Core Data for Automotive Mechanical Design Process');
#67053=PRODUCT_CONTEXT('part definition',#67052,'mechanical');
#67084=PRODUCT('Coupling Hub 2','Coupling Hub 2',$,(#67053));
#67095=PRESENTATION_STYLE_ASSIGNMENT((#67097));
#67097=SURFACE_STYLE_USAGE(.BOTH.,#67099);
#67099=SURFACE_SIDE_STYLE('',(#67101));
#67101=SURFACE_STYLE_FILL_AREA(#67103);
#67103=FILL_AREA_STYLE('Opaque(202,209,238)',(#67105));
#67105=FILL_AREA_STYLE_COLOUR('Opaque(202,209,238)',#67107);
#67107=COLOUR_RGB('Opaque(202,209,238)',0.792156862745098,0.819607843137255,
0.933333333333333);
ENDSEC;
END-ISO-10303-21;
